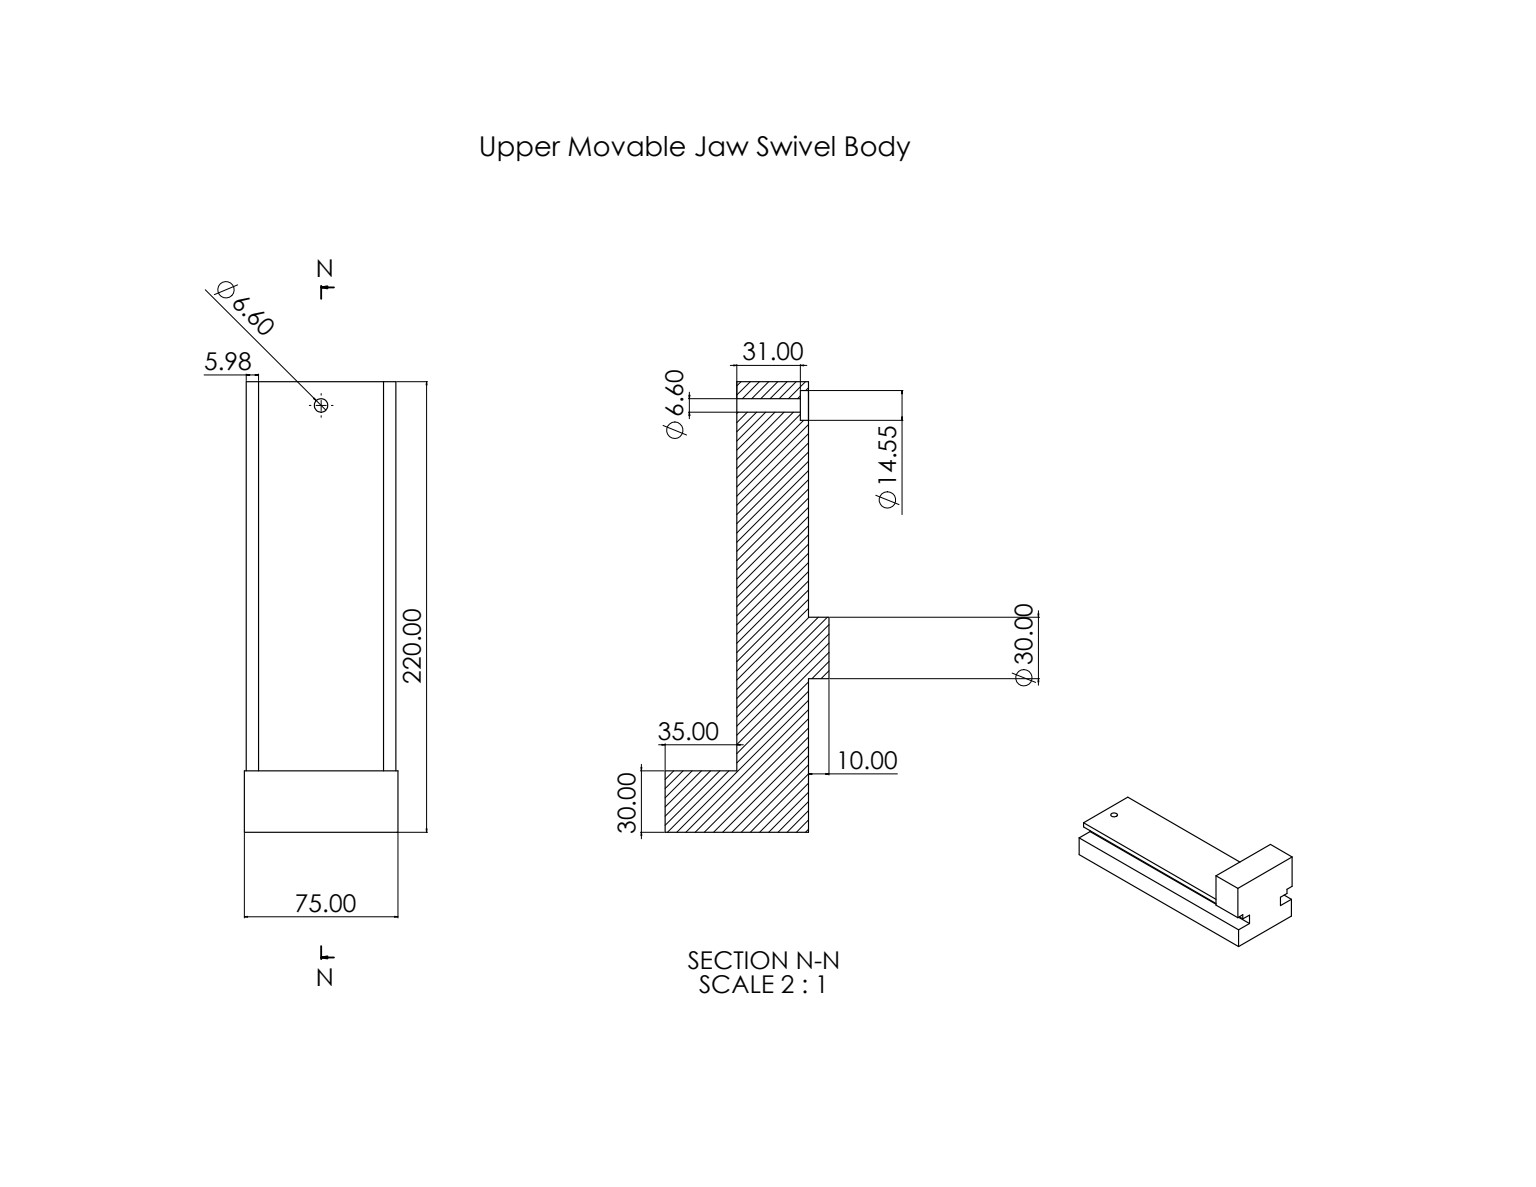
ISO-10303-21;
HEADER;
FILE_DESCRIPTION (('STEP AP214'),
    '1' );
FILE_NAME ('Upper Movable Jaw Swivel Body.step',
    '2026-10-24T22:31:37',
    ( '' ),
    ( '' ),
    'SwSTEP 2.0',
    'SolidWorks 2025',
    '' );
FILE_SCHEMA (( 'AUTOMOTIVE_DESIGN' ));
ENDSEC;

DATA;
#88=ORIENTED_EDGE ( 'NONE', *, *, #97854, .T. ) ;
#107=CARTESIAN_POINT ( 'NONE',  ( -32.94356256989595977, 94.88921800892812541, 10.61543114587583503 ) ) ;
#112=EDGE_CURVE ( 'NONE', #27867, #86369, #27228, .T. ) ;
#449=DIRECTION ( 'NONE',  ( 0.8660254037844391517, 0.4999999999999990008, 0.000000000000000000 ) ) ;
#471=DIRECTION ( 'NONE',  ( 0.8660254037844373753, 0.5000000000000021094, 0.000000000000000000 ) ) ;
#478=CARTESIAN_POINT ( 'NONE',  ( -32.68486601307109396, 95.73265939123938040, 11.22505256784756611 ) ) ;
#599=DIRECTION ( 'NONE',  ( 0.8660254037844382635, 0.5000000000000005551, 0.000000000000000000 ) ) ;
#606=VECTOR ( 'NONE', #83343, 1000.000000000000114 ) ;
#639=PLANE ( 'NONE',  #90141 ) ;
#678=( LENGTH_UNIT ( ) NAMED_UNIT ( * ) SI_UNIT ( .MILLI., .METRE. ) );
#987=ORIENTED_EDGE ( 'NONE', *, *, #63428, .F. ) ;
#1016=CARTESIAN_POINT ( 'NONE',  ( 77.93017357788673394, 184.0458036431182052, -30.52142883766498116 ) ) ;
#1096=DIRECTION ( 'NONE',  ( 0.000000000000000000, 0.000000000000000000, 1.000000000000000000 ) ) ;
#1182=DIRECTION ( 'NONE',  ( 0.8660254037844382635, 0.5000000000000005551, 0.000000000000000000 ) ) ;
#1406=VECTOR ( 'NONE', #11738, 1000.000000000000000 ) ;
#1495=ORIENTED_EDGE ( 'NONE', *, *, #73193, .T. ) ;
#1508=ORIENTED_EDGE ( 'NONE', *, *, #88243, .F. ) ;
#1527=ORIENTED_EDGE ( 'NONE', *, *, #76895, .F. ) ;
#1594=CARTESIAN_POINT ( 'NONE',  ( -167.0327448629461742, 42.61639673982678289, 21.50000000000000000 ) ) ;
#1831=ORIENTED_EDGE ( 'NONE', *, *, #24685, .F. ) ;
#2126=VERTEX_POINT ( 'NONE', #95140 ) ;
#2173=CARTESIAN_POINT ( 'NONE',  ( -132.5954152546898115, 108.6868197944956478, 37.50000000000002132 ) ) ;
#2180=DIRECTION ( 'NONE',  ( 1.000000000000000000, 0.000000000000000000, 0.000000000000000000 ) ) ;
#2356=CARTESIAN_POINT ( 'NONE',  ( -107.5954152546897262, 65.38554960527366688, -21.50000000000000000 ) ) ;
#2371=ORIENTED_EDGE ( 'NONE', *, *, #69900, .T. ) ;
#2442=CARTESIAN_POINT ( 'NONE',  ( -31.55997627504339320, 93.43085135866357405, 11.06573829301134282 ) ) ;
#2563=FACE_OUTER_BOUND ( 'NONE', #81678, .T. ) ;
#2588=EDGE_CURVE ( 'NONE', #83357, #20667, #32841, .T. ) ;
#2781=VECTOR ( 'NONE', #47717, 1000.000000000000227 ) ;
#2784=UNCERTAINTY_MEASURE_WITH_UNIT (LENGTH_MEASURE( 1.000000000000000082E-05 ), #94636, 'distance_accuracy_value', 'NONE');
#3036=VECTOR ( 'NONE', #61789, 1000.000000000000000 ) ;
#3092=ORIENTED_EDGE ( 'NONE', *, *, #37488, .F. ) ;
#3134=VECTOR ( 'NONE', #87868, 1000.000000000000000 ) ;
#3372=CARTESIAN_POINT ( 'NONE',  ( 65.36586985908989789, 182.5653022007868742, 0.000000000000000000 ) ) ;
#3536=DIRECTION ( 'NONE',  ( 0.5000000000000002220, -0.8660254037844387076, -0.000000000000000000 ) ) ;
#3607=CARTESIAN_POINT ( 'NONE',  ( -32.02765978341597730, 96.24804957567249630, 11.90709431551868214 ) ) ;
#3843=ORIENTED_EDGE ( 'NONE', *, *, #39130, .F. ) ;
#3870=ORIENTED_EDGE ( 'NONE', *, *, #76643, .F. ) ;
#3921=CARTESIAN_POINT ( 'NONE',  ( -32.85596848784926038, 94.38113866725780099, 10.43451941826970319 ) ) ;
#3932=ORIENTED_EDGE ( 'NONE', *, *, #2588, .T. ) ;
#4006=VECTOR ( 'NONE', #42693, 1000.000000000000000 ) ;
#4058=DIRECTION ( 'NONE',  ( 0.000000000000000000, 0.000000000000000000, -1.000000000000000000 ) ) ;
#4066=LINE ( 'NONE', #89237, #62676 ) ;
#4351=CARTESIAN_POINT ( 'NONE',  ( -14.30703472742949245, 105.2809231865207522, 10.47389102980036313 ) ) ;
#4594=LINE ( 'NONE', #12204, #86850 ) ;
#4680=CYLINDRICAL_SURFACE ( 'NONE', #36010, 3.300000000000010925 ) ;
#4830=VECTOR ( 'NONE', #48570, 1000.000000000000227 ) ;
#4863=ORIENTED_EDGE ( 'NONE', *, *, #15300, .T. ) ;
#4920=CARTESIAN_POINT ( 'NONE',  ( -13.86269525828469895, 104.2312461070084879, 10.61543114587583148 ) ) ;
#5067=FACE_OUTER_BOUND ( 'NONE', #46254, .T. ) ;
#5071=ORIENTED_EDGE ( 'NONE', *, *, #58498, .F. ) ;
#5089=DIRECTION ( 'NONE',  ( 0.8660254037844385966, 0.5000000000000001110, -0.000000000000000000 ) ) ;
#5122=LINE ( 'NONE', #90768, #6948 ) ;
#5352=CARTESIAN_POINT ( 'NONE',  ( -14.46602979551751389, 105.4129113170957481, 10.54689744722228006 ) ) ;
#5376=FACE_OUTER_BOUND ( 'NONE', #49831, .T. ) ;
#5390=VECTOR ( 'NONE', #56746, 1000.000000000000114 ) ;
#5468=ORIENTED_EDGE ( 'NONE', *, *, #67897, .F. ) ;
#5479=ADVANCED_FACE ( 'NONE', ( #20384 ), #4680, .F. ) ;
#5488=CARTESIAN_POINT ( 'NONE',  ( -167.0327448629461742, 42.61639673982678289, -21.50000000000000000 ) ) ;
#5508=CARTESIAN_POINT ( 'NONE',  ( 80.86586985908986946, 155.7185146834693512, 0.000000000000000000 ) ) ;
#5738=CARTESIAN_POINT ( 'NONE',  ( -14.65312891409034535, 84.40478749174073414, 0.000000000000000000 ) ) ;
#5800=FACE_OUTER_BOUND ( 'NONE', #65592, .T. ) ;
#5844=CARTESIAN_POINT ( 'NONE',  ( -16.76269525828470464, 104.2312461070085021, 12.63376007436041171 ) ) ;
#5851=DIRECTION ( 'NONE',  ( -0.000000000000000000, -0.000000000000000000, 1.000000000000000000 ) ) ;
#5871=PLANE ( 'NONE',  #22534 ) ;
#5896=ADVANCED_FACE ( 'NONE', ( #7535 ), #53628, .F. ) ;
#5923=ORIENTED_EDGE ( 'NONE', *, *, #44335, .T. ) ;
#5975=AXIS2_PLACEMENT_3D ( 'NONE', #18174, #69859, #471 ) ;
#6124=CIRCLE ( 'NONE', #70862, 7.273499999999997634 ) ;
#6152=FACE_OUTER_BOUND ( 'NONE', #19578, .T. ) ;
#6375=ADVANCED_FACE ( 'NONE', ( #54494 ), #23602, .T. ) ;
#6428=CONICAL_SURFACE ( 'NONE', #56528, 7.298499999999999766, 0.7853981633976494514 ) ;
#6948=VECTOR ( 'NONE', #7990, 1000.000000000000000 ) ;
#7015=ORIENTED_EDGE ( 'NONE', *, *, #33038, .F. ) ;
#7114=CARTESIAN_POINT ( 'NONE',  ( -97.59541525468981149, 48.06504152958505216, 36.50000000000000000 ) ) ;
#7240=VECTOR ( 'NONE', #599, 1000.000000000000114 ) ;
#7282=CARTESIAN_POINT ( 'NONE',  ( -27.64350997085663408, 76.90478749174087625, 0.000000000000000000 ) ) ;
#7348=VERTEX_POINT ( 'NONE', #39001 ) ;
#7439=ORIENTED_EDGE ( 'NONE', *, *, #88245, .T. ) ;
#7459=CARTESIAN_POINT ( 'NONE',  ( 82.93017357788667709, 175.3855496052738374, 36.50000000000000000 ) ) ;
#7460=DIRECTION ( 'NONE',  ( -0.000000000000000000, -0.000000000000000000, -1.000000000000000000 ) ) ;
#7523=ORIENTED_EDGE ( 'NONE', *, *, #37488, .T. ) ;
#7535=FACE_OUTER_BOUND ( 'NONE', #52527, .T. ) ;
#7609=LINE ( 'NONE', #1016, #16237 ) ;
#7691=DIRECTION ( 'NONE',  ( 0.5000000000000000000, -0.8660254037844387076, 0.000000000000000000 ) ) ;
#7767=VECTOR ( 'NONE', #54858, 1000.000000000000114 ) ;
#7861=EDGE_LOOP ( 'NONE', ( #9188, #92716, #77192, #81964 ) ) ;
#7990=DIRECTION ( 'NONE',  ( 0.4999999999999985012, -0.8660254037844394848, -1.387778780781440351E-15 ) ) ;
#8389=DIRECTION ( 'NONE',  ( -0.000000000000000000, -0.000000000000000000, 1.000000000000000000 ) ) ;
#8417=CARTESIAN_POINT ( 'NONE',  ( -89.11465314115667979, 93.37593066204033221, -30.52142883766496695 ) ) ;
#8555=CARTESIAN_POINT ( 'NONE',  ( 74.56683408466376761, 152.0817646834693448, 8.907468493598274475E-16 ) ) ;
#8757=LINE ( 'NONE', #2173, #11074 ) ;
#8809=ORIENTED_EDGE ( 'NONE', *, *, #62129, .T. ) ;
#8849=EDGE_LOOP ( 'NONE', ( #90481, #9070, #75347, #22436 ) ) ;
#8886=DIRECTION ( 'NONE',  ( -0.5000000000000003331, 0.8660254037844383745, 0.000000000000000000 ) ) ;
#8976=CARTESIAN_POINT ( 'NONE',  ( -106.6146531411566798, 123.6868197944956620, 37.50000000000002132 ) ) ;
#9070=ORIENTED_EDGE ( 'NONE', *, *, #32666, .F. ) ;
#9078=DIRECTION ( 'NONE',  ( 0.8660254037844384856, 0.5000000000000002220, 0.000000000000000000 ) ) ;
#9152=ORIENTED_EDGE ( 'NONE', *, *, #45013, .T. ) ;
#9188=ORIENTED_EDGE ( 'NONE', *, *, #12031, .F. ) ;
#9235=AXIS2_PLACEMENT_3D ( 'NONE', #17271, #24379, #9699 ) ;
#9406=ORIENTED_EDGE ( 'NONE', *, *, #12031, .T. ) ;
#9506=ADVANCED_FACE ( 'NONE', ( #29685 ), #76775, .T. ) ;
#9510=LINE ( 'NONE', #71312, #77599 ) ;
#9699=DIRECTION ( 'NONE',  ( 0.8660254037844373753, 0.5000000000000021094, 0.000000000000000000 ) ) ;
#9759=EDGE_CURVE ( 'NONE', #12458, #43772, #86395, .T. ) ;
#9788=CARTESIAN_POINT ( 'NONE',  ( -169.5327448629461742, 46.94652375874896677, 30.52142883766498827 ) ) ;
#9801=SHAPE_REPRESENTATION_RELATIONSHIP ( 'NONE' , 'NONE' ,  #87244, #17532 ) ;
#10026=CARTESIAN_POINT ( 'NONE',  ( 77.93017357788673394, 184.0458036431182052, 21.50000000000000000 ) ) ;
#10028=ORIENTED_EDGE ( 'NONE', *, *, #69900, .F. ) ;
#10091=DIRECTION ( 'NONE',  ( 0.5000000000000005551, -0.8660254037844382635, -3.965082230804119373E-16 ) ) ;
#10101=DIRECTION ( 'NONE',  ( 0.8660254037844382635, 0.5000000000000005551, 0.000000000000000000 ) ) ;
#10174=EDGE_CURVE ( 'NONE', #37839, #84449, #78305, .T. ) ;
#10179=DIRECTION ( 'NONE',  ( -0.8660254037844375974, -0.5000000000000016653, 0.000000000000000000 ) ) ;
#10198=EDGE_CURVE ( 'NONE', #33624, #79062, #80847, .T. ) ;
#10307=FACE_OUTER_BOUND ( 'NONE', #41949, .T. ) ;
#10553=ORIENTED_EDGE ( 'NONE', *, *, #33693, .T. ) ;
#10719=PLANE ( 'NONE',  #41218 ) ;
#10723=EDGE_LOOP ( 'NONE', ( #84176, #16172 ) ) ;
#10803=VERTEX_POINT ( 'NONE', #67448 ) ;
#10818=CARTESIAN_POINT ( 'NONE',  ( -107.5954152546898257, 65.38554960527383741, 36.50000000000000000 ) ) ;
#10849=ADVANCED_FACE ( 'NONE', ( #75563, #6152 ), #37045, .F. ) ;
#10855=CYLINDRICAL_SURFACE ( 'NONE', #91491, 14.99999999999968381 ) ;
#11014=VECTOR ( 'NONE', #31568, 1000.000000000000000 ) ;
#11074=VECTOR ( 'NONE', #17874, 1000.000000000000000 ) ;
#11139=DIRECTION ( 'NONE',  ( 0.5000000000000001110, -0.8660254037844384856, -0.000000000000000000 ) ) ;
#11216=CARTESIAN_POINT ( 'NONE',  ( -31.49991166888935368, 96.34225309604657639, 12.27547638658930218 ) ) ;
#11235=CARTESIAN_POINT ( 'NONE',  ( -167.0327448629461742, 42.61639673982675447, 30.52142883766498116 ) ) ;
#11374=AXIS2_PLACEMENT_3D ( 'NONE', #37260, #99085, #91499 ) ;
#11419=DIRECTION ( 'NONE',  ( -0.5000000000000002220, 0.8660254037844384856, 1.387778780781440548E-15 ) ) ;
#11527=CARTESIAN_POINT ( 'NONE',  ( -112.5954152546897120, 74.04580364311804885, -30.52142883766498116 ) ) ;
#11529=CARTESIAN_POINT ( 'NONE',  ( -16.75143828124104317, 104.0219442184326937, 12.69405866495271695 ) ) ;
#11540=CARTESIAN_POINT ( 'NONE',  ( -30.74734981195323158, 93.63450014558806345, 11.75270985346817909 ) ) ;
#11738=DIRECTION ( 'NONE',  ( -0.000000000000000000, -0.000000000000000000, 1.000000000000000000 ) ) ;
#11834=CARTESIAN_POINT ( 'NONE',  ( 82.93017357788673394, 175.3855496052738374, 21.50000000000000000 ) ) ;
#11858=CARTESIAN_POINT ( 'NONE',  ( 82.85336985908988083, 152.2760637034261890, 0.000000000000000000 ) ) ;
#11912=CARTESIAN_POINT ( 'NONE',  ( 76.55433408466377898, 148.6393137034262111, 8.907468493598274475E-16 ) ) ;
#11989=PRODUCT_DEFINITION_SHAPE ( 'NONE', 'NONE',  #32837 ) ;
#12018=CARTESIAN_POINT ( 'NONE',  ( -16.52110513491133759, 103.4226009623137514, 12.75654370805655091 ) ) ;
#12031=EDGE_CURVE ( 'NONE', #10803, #33624, #9510, .T. ) ;
#12050=CARTESIAN_POINT ( 'NONE',  ( 89.15240563351599690, 155.9128137034261954, 0.000000000000000000 ) ) ;
#12170=CARTESIAN_POINT ( 'NONE',  ( 82.93017357788673394, 175.3855496052738374, -21.50000000000000000 ) ) ;
#12198=CARTESIAN_POINT ( 'NONE',  ( -30.22813246154364109, 95.60533857986700923, 12.75846431767311451 ) ) ;
#12204=CARTESIAN_POINT ( 'NONE',  ( -89.11465314115667979, 93.37593066204033221, -30.52142883766496695 ) ) ;
#12217=DIRECTION ( 'NONE',  ( 0.000000000000000000, -1.000000000000000000, -1.201851678989722492E-15 ) ) ;
#12458=VERTEX_POINT ( 'NONE', #69665 ) ;
#12466=CARTESIAN_POINT ( 'NONE',  ( -15.24570502058241139, 105.6897125274499842, 11.06526020485377160 ) ) ;
#12473=CYLINDRICAL_SURFACE ( 'NONE', #44723, 1.449999999999993072 ) ;
#12517=CARTESIAN_POINT ( 'NONE',  ( -14.03049543618944206, 103.5316844796765565, 11.08926661400182390 ) ) ;
#12561=ORIENTED_EDGE ( 'NONE', *, *, #34818, .T. ) ;
#12682=DIRECTION ( 'NONE',  ( -0.5000000000000008882, 0.8660254037844381525, 0.000000000000000000 ) ) ;
#12687=AXIS2_PLACEMENT_3D ( 'NONE', #69833, #100261, #59733 ) ;
#12698=LINE ( 'NONE', #73992, #85196 ) ;
#12974=CARTESIAN_POINT ( 'NONE',  ( -15.07180212829954158, 105.6728077113080673, 10.93289567214266711 ) ) ;
#12998=CARTESIAN_POINT ( 'NONE',  ( -30.04356256989597185, 94.88921800892812541, 36.50000000000000000 ) ) ;
#13058=CARTESIAN_POINT ( 'NONE',  ( 87.16490563351598553, 159.3552646834693292, 0.000000000000000000 ) ) ;
#13093=EDGE_LOOP ( 'NONE', ( #90102, #1495, #15262, #82142 ) ) ;
#13128=LINE ( 'NONE', #14612, #83498 ) ;
#13202=CARTESIAN_POINT ( 'NONE',  ( -30.10073558955866702, 95.30624366923747459, 12.73418565006493175 ) ) ;
#13422=DIRECTION ( 'NONE',  ( 1.000000000000000000, 0.000000000000000000, 0.000000000000000000 ) ) ;
#13483=EDGE_LOOP ( 'NONE', ( #22501, #42882, #25014, #81312 ) ) ;
#13558=VECTOR ( 'NONE', #32477, 1000.000000000000114 ) ;
#13570=AXIS2_PLACEMENT_3D ( 'NONE', #14550, #53030, #65862 ) ;
#13616=DIRECTION ( 'NONE',  ( 0.5000000000000002220, -0.8660254037844387076, -0.000000000000000000 ) ) ;
#13794=ORIENTED_EDGE ( 'NONE', *, *, #88245, .F. ) ;
#14075=DIRECTION ( 'NONE',  ( 0.5000000000000006661, -0.8660254037844383745, -3.433594394091488070E-15 ) ) ;
#14147=VECTOR ( 'NONE', #8389, 1000.000000000000000 ) ;
#14187=CARTESIAN_POINT ( 'NONE',  ( -32.32883188359665638, 96.08671883726218255, 11.63744038197175534 ) ) ;
#14193=CARTESIAN_POINT ( 'NONE',  ( -32.94356256989595977, 94.88921800892812541, 36.50000000000000000 ) ) ;
#14304=AXIS2_PLACEMENT_3D ( 'NONE', #83231, #7691, #67996 ) ;
#14470=DIRECTION ( 'NONE',  ( 0.000000000000000000, 0.000000000000000000, 1.000000000000000000 ) ) ;
#14550=CARTESIAN_POINT ( 'NONE',  ( -15.31269525828471068, 104.2312461070085021, 36.50000000000000000 ) ) ;
#14566=EDGE_LOOP ( 'NONE', ( #92678, #83072, #30486, #36692 ) ) ;
#14612=CARTESIAN_POINT ( 'NONE',  ( -106.6146531411566798, 123.6868197944956620, 37.50000000000002132 ) ) ;
#14681=CARTESIAN_POINT ( 'NONE',  ( -32.77609386396424185, 95.58753423100951352, 11.08839328151203851 ) ) ;
#14906=ORIENTED_EDGE ( 'NONE', *, *, #33038, .T. ) ;
#15085=DIRECTION ( 'NONE',  ( 0.000000000000000000, -0.000000000000000000, 1.000000000000000000 ) ) ;
#15251=LINE ( 'NONE', #1594, #13558 ) ;
#15262=ORIENTED_EDGE ( 'NONE', *, *, #99216, .F. ) ;
#15267=CARTESIAN_POINT ( 'NONE',  ( 0.000000000000000000, 0.000000000000000000, -36.50000000000000000 ) ) ;
#15300=EDGE_CURVE ( 'NONE', #94383, #88861, #37826, .T. ) ;
#15314=ADVANCED_FACE ( 'NONE', ( #37879 ), #22709, .T. ) ;
#15354=CARTESIAN_POINT ( 'NONE',  ( 0.000000000000000000, 0.000000000000000000, 0.000000000000000000 ) ) ;
#15546=PLANE ( 'NONE',  #96769 ) ;
#15668=ORIENTED_EDGE ( 'NONE', *, *, #91252, .F. ) ;
#15713=CYLINDRICAL_SURFACE ( 'NONE', #61431, 1.449999999999993072 ) ;
#15866=AXIS2_PLACEMENT_3D ( 'NONE', #15267, #1096, #69484 ) ;
#15879=VECTOR ( 'NONE', #30098, 999.9999999999998863 ) ;
#15919=VECTOR ( 'NONE', #98723, 1000.000000000000000 ) ;
#16027=ORIENTED_EDGE ( 'NONE', *, *, #57557, .F. ) ;
#16172=ORIENTED_EDGE ( 'NONE', *, *, #9759, .T. ) ;
#16182=VECTOR ( 'NONE', #99200, 1000.000000000000114 ) ;
#16237=VECTOR ( 'NONE', #47103, 1000.000000000000114 ) ;
#16312=CARTESIAN_POINT ( 'NONE',  ( -1.662747857324051282, 91.90478749174060624, 1.836970198720990540E-15 ) ) ;
#16329=LINE ( 'NONE', #78145, #88768 ) ;
#16549=CARTESIAN_POINT ( 'NONE',  ( -169.5327448629461742, 46.94652375874896677, 30.52142883766498827 ) ) ;
#16698=ORIENTED_EDGE ( 'NONE', *, *, #50936, .F. ) ;
#16721=EDGE_CURVE ( 'NONE', #7348, #56899, #5122, .T. ) ;
#16855=VECTOR ( 'NONE', #32280, 1000.000000000000114 ) ;
#16871=LINE ( 'NONE', #40156, #51977 ) ;
#17082=ADVANCED_FACE ( 'NONE', ( #44850 ), #61041, .T. ) ;
#17173=ORIENTED_EDGE ( 'NONE', *, *, #45138, .F. ) ;
#17200=VECTOR ( 'NONE', #22885, 1000.000000000000000 ) ;
#17265=ORIENTED_EDGE ( 'NONE', *, *, #17424, .T. ) ;
#17271=CARTESIAN_POINT ( 'NONE',  ( 80.86586985908986946, 155.7185146834693512, 0.000000000000000000 ) ) ;
#17365=ADVANCED_FACE ( 'NONE', ( #62930 ), #639, .T. ) ;
#17424=EDGE_CURVE ( 'NONE', #27867, #82530, #25430, .T. ) ;
#17532=ADVANCED_BREP_SHAPE_REPRESENTATION ( '', ( #77374, #68784 ), #36458 ) ;
#17765=CARTESIAN_POINT ( 'NONE',  ( -167.0327448629461742, 42.61639673982678289, -21.50000000000000000 ) ) ;
#17787=EDGE_LOOP ( 'NONE', ( #74842, #9152, #46683, #35102 ) ) ;
#17874=DIRECTION ( 'NONE',  ( -7.401486830834377265E-16, 7.401486830834377265E-16, -1.000000000000000000 ) ) ;
#17933=AXIS2_PLACEMENT_3D ( 'NONE', #67594, #82850, #74235 ) ;
#18128=CARTESIAN_POINT ( 'NONE',  ( -30.04356256989558815, 94.88921800892795488, 12.63376007436073323 ) ) ;
#18174=CARTESIAN_POINT ( 'NONE',  ( 80.86586985908986946, 155.7185146834693512, 0.000000000000000000 ) ) ;
#18282=EDGE_CURVE ( 'NONE', #99384, #50939, #27437, .T. ) ;
#18412=ORIENTED_EDGE ( 'NONE', *, *, #86727, .F. ) ;
#18517=EDGE_CURVE ( 'NONE', #23627, #46799, #73912, .T. ) ;
#18560=DIRECTION ( 'NONE',  ( -1.982541115402060426E-16, 3.433861939970638790E-16, -1.000000000000000000 ) ) ;
#18566=DIRECTION ( 'NONE',  ( 0.8660254037844377084, 0.5000000000000016653, 0.000000000000000000 ) ) ;
#18568=CARTESIAN_POINT ( 'NONE',  ( -16.56403295706242318, 104.9882471913986990, 12.26538863783448186 ) ) ;
#18579=ORIENTED_EDGE ( 'NONE', *, *, #93323, .T. ) ;
#18690=ORIENTED_EDGE ( 'NONE', *, *, #57557, .T. ) ;
#18827=APPLICATION_CONTEXT ( 'automotive_design' ) ;
#18886=CARTESIAN_POINT ( 'NONE',  ( -13.86269525828469895, 104.2312461070084879, 10.61543114587583148 ) ) ;
#18947=LINE ( 'NONE', #49826, #33470 ) ;
#19147=CARTESIAN_POINT ( 'NONE',  ( -30.24407882362163846, 94.12867598954146331, 12.26304263616266077 ) ) ;
#19442=ORIENTED_EDGE ( 'NONE', *, *, #68029, .F. ) ;
#19531=ORIENTED_EDGE ( 'NONE', *, *, #89878, .F. ) ;
#19560=DIRECTION ( 'NONE',  ( 0.5000000000000001110, -0.8660254037844384856, -0.000000000000000000 ) ) ;
#19578=EDGE_LOOP ( 'NONE', ( #4863, #88 ) ) ;
#19581=CARTESIAN_POINT ( 'NONE',  ( -14.23124088391897146, 105.2031859152619120, 10.44627079400605218 ) ) ;
#19596=EDGE_CURVE ( 'NONE', #91708, #27867, #13128, .T. ) ;
#19632=CARTESIAN_POINT ( 'NONE',  ( -16.31118285231257303, 103.1745050122371481, 12.72070314857826467 ) ) ;
#19643=CARTESIAN_POINT ( 'NONE',  ( -30.60512737934784155, 93.72946926685976621, 11.88605707516453691 ) ) ;
#19824=ORIENTED_EDGE ( 'NONE', *, *, #67897, .T. ) ;
#19825=CARTESIAN_POINT ( 'NONE',  ( 82.93017357788667709, 175.3855496052738374, 36.50000000000000000 ) ) ;
#19890=DIRECTION ( 'NONE',  ( 0.8660254037844373753, 0.5000000000000021094, 0.000000000000000000 ) ) ;
#19964=VERTEX_POINT ( 'NONE', #44378 ) ;
#20066=CARTESIAN_POINT ( 'NONE',  ( -14.55094619507370801, 105.4688078659398514, 10.59293022331821099 ) ) ;
#20069=DIRECTION ( 'NONE',  ( -0.8660254037844382635, -0.5000000000000004441, 0.000000000000000000 ) ) ;
#20118=CARTESIAN_POINT ( 'NONE',  ( -14.76680962501131589, 102.8402364515597469, 11.91671626263131856 ) ) ;
#20129=CARTESIAN_POINT ( 'NONE',  ( -32.26013835757641601, 93.64104699330448511, 10.58366280279360971 ) ) ;
#20179=DIRECTION ( 'NONE',  ( 0.5000000000000014433, -0.8660254037844379305, 0.000000000000000000 ) ) ;
#20243=DIRECTION ( 'NONE',  ( 0.8660254037844391517, 0.4999999999999990008, 0.000000000000000000 ) ) ;
#20307=ORIENTED_EDGE ( 'NONE', *, *, #86286, .T. ) ;
#20384=FACE_OUTER_BOUND ( 'NONE', #17787, .T. ) ;
#20667=VERTEX_POINT ( 'NONE', #58531 ) ;
#20988=EDGE_CURVE ( 'NONE', #84449, #47085, #84745, .T. ) ;
#21072=ORIENTED_EDGE ( 'NONE', *, *, #77053, .T. ) ;
#21291=LINE ( 'NONE', #35969, #67737 ) ;
#21354=EDGE_CURVE ( 'NONE', #62277, #32844, #96223, .T. ) ;
#21790=AXIS2_PLACEMENT_3D ( 'NONE', #73940, #67832, #20243 ) ;
#21893=LINE ( 'NONE', #98918, #17200 ) ;
#22006=ORIENTED_EDGE ( 'NONE', *, *, #21354, .F. ) ;
#22032=CARTESIAN_POINT ( 'NONE',  ( -16.76269525828470464, 104.4383445782105042, 12.56748295067274945 ) ) ;
#22180=VECTOR ( 'NONE', #42070, 1000.000000000000114 ) ;
#22397=ORIENTED_EDGE ( 'NONE', *, *, #41041, .F. ) ;
#22436=ORIENTED_EDGE ( 'NONE', *, *, #95215, .T. ) ;
#22501=ORIENTED_EDGE ( 'NONE', *, *, #23408, .F. ) ;
#22522=VECTOR ( 'NONE', #62854, 1000.000000000000000 ) ;
#22526=VECTOR ( 'NONE', #1182, 1000.000000000000114 ) ;
#22534=AXIS2_PLACEMENT_3D ( 'NONE', #98595, #14470, #68652 ) ;
#22639=EDGE_LOOP ( 'NONE', ( #58236, #64858, #7523, #3843 ) ) ;
#22709=PLANE ( 'NONE',  #89665 ) ;
#22835=EDGE_CURVE ( 'NONE', #85740, #37839, #63017, .T. ) ;
#22880=FACE_OUTER_BOUND ( 'NONE', #67161, .T. ) ;
#22885=DIRECTION ( 'NONE',  ( -0.2588190451027150840, -0.9659258262890161317, 8.659560562356675748E-17 ) ) ;
#22966=( NAMED_UNIT ( * ) SI_UNIT ( $, .STERADIAN. ) SOLID_ANGLE_UNIT ( ) );
#23131=CARTESIAN_POINT ( 'NONE',  ( -89.11465314115662295, 93.37593066204024694, -30.52142883766498116 ) ) ;
#23363=EDGE_LOOP ( 'NONE', ( #18412, #51644, #99432, #18690 ) ) ;
#23373=LINE ( 'NONE', #77608, #70923 ) ;
#23390=CARTESIAN_POINT ( 'NONE',  ( 82.93017357788667709, 175.3855496052738374, 36.50000000000000000 ) ) ;
#23408=EDGE_CURVE ( 'NONE', #98986, #24620, #81400, .T. ) ;
#23457=DIRECTION ( 'NONE',  ( 1.000000000000000000, 0.000000000000000000, 0.000000000000000000 ) ) ;
#23602=PLANE ( 'NONE',  #67693 ) ;
#23608=EDGE_LOOP ( 'NONE', ( #8809, #13794, #86714, #37581, #78724, #9406, #80355, #86475, #67151, #79423, #31254, #86823, #5923, #41180, #92068, #80132 ) ) ;
#23627=VERTEX_POINT ( 'NONE', #89514 ) ;
#23629=CARTESIAN_POINT ( 'NONE',  ( 62.50798602660126591, 180.9153022007868685, 4.041334437186263538E-16 ) ) ;
#23630=ADVANCED_FACE ( 'NONE', ( #81896 ), #12473, .F. ) ;
#23875=PLANE ( 'NONE',  #15866 ) ;
#23896=DIRECTION ( 'NONE',  ( -0.8660254037844385966, -0.4999999999999999445, 0.000000000000000000 ) ) ;
#23972=VERTEX_POINT ( 'NONE', #34847 ) ;
#24157=PLANE ( 'NONE',  #43501 ) ;
#24326=DIRECTION ( 'NONE',  ( 0.5000000000000000000, -0.8660254037844387076, 0.000000000000000000 ) ) ;
#24373=ORIENTED_EDGE ( 'NONE', *, *, #40599, .F. ) ;
#24379=DIRECTION ( 'NONE',  ( 0.5000000000000002220, -0.8660254037844387076, -0.000000000000000000 ) ) ;
#24447=EDGE_LOOP ( 'NONE', ( #93056, #65035 ) ) ;
#24486=AXIS2_PLACEMENT_3D ( 'NONE', #99117, #29699, #45388 ) ;
#24620=VERTEX_POINT ( 'NONE', #81268 ) ;
#24685=EDGE_CURVE ( 'NONE', #67744, #41262, #18947, .T. ) ;
#24700=CARTESIAN_POINT ( 'NONE',  ( -89.11465314115665137, 93.37593066204027537, 37.50000000000002132 ) ) ;
#24766=PLANE ( 'NONE',  #43274 ) ;
#24982=ORIENTED_EDGE ( 'NONE', *, *, #29271, .F. ) ;
#25014=ORIENTED_EDGE ( 'NONE', *, *, #41013, .F. ) ;
#25049=PRODUCT_DEFINITION_CONTEXT ( 'detailed design', #54587, 'design' ) ;
#25103=ORIENTED_EDGE ( 'NONE', *, *, #86286, .F. ) ;
#25219=CARTESIAN_POINT ( 'NONE',  ( -97.59541525468981149, 48.06504152958505216, 36.50000000000000000 ) ) ;
#25232=ORIENTED_EDGE ( 'NONE', *, *, #59302, .F. ) ;
#25430=LINE ( 'NONE', #47230, #2781 ) ;
#25626=ADVANCED_FACE ( 'NONE', ( #50332 ), #10855, .T. ) ;
#25654=CIRCLE ( 'NONE', #48349, 3.299999999999998934 ) ;
#25739=CARTESIAN_POINT ( 'NONE',  ( -32.76508427577140736, 94.18386203199597162, 10.41389758979254587 ) ) ;
#25748=ORIENTED_EDGE ( 'NONE', *, *, #94596, .F. ) ;
#26009=ORIENTED_EDGE ( 'NONE', *, *, #34192, .T. ) ;
#26014=DIRECTION ( 'NONE',  ( 0.5000000000000001110, -0.8660254037844385966, 0.000000000000000000 ) ) ;
#26521=VERTEX_POINT ( 'NONE', #46463 ) ;
#26564=FACE_OUTER_BOUND ( 'NONE', #46792, .T. ) ;
#26953=CARTESIAN_POINT ( 'NONE',  ( -107.5954152546898257, 65.38554960527383741, -21.50000000000000000 ) ) ;
#27228=LINE ( 'NONE', #41405, #92812 ) ;
#27229=CARTESIAN_POINT ( 'NONE',  ( -32.94356256989596687, 94.79146141117595903, 10.56663419031904638 ) ) ;
#27437=LINE ( 'NONE', #81173, #1406 ) ;
#27607=ORIENTED_EDGE ( 'NONE', *, *, #83276, .T. ) ;
#27638=ORIENTED_EDGE ( 'NONE', *, *, #39847, .F. ) ;
#27645=LINE ( 'NONE', #35724, #48129 ) ;
#27666=CARTESIAN_POINT ( 'NONE',  ( -13.95001416935992289, 104.7385778355855592, 10.43465946748403184 ) ) ;
#27867=VERTEX_POINT ( 'NONE', #89401 ) ;
#27902=ORIENTED_EDGE ( 'NONE', *, *, #34818, .F. ) ;
#28141=CARTESIAN_POINT ( 'NONE',  ( 83.72375369157853697, 157.3685146834693569, 0.000000000000000000 ) ) ;
#28296=DIRECTION ( 'NONE',  ( 0.8660254037844390407, 0.4999999999999993339, 0.000000000000000000 ) ) ;
#28683=DIRECTION ( 'NONE',  ( 0.8660254037844384856, 0.5000000000000002220, 0.000000000000000000 ) ) ;
#28818=EDGE_CURVE ( 'NONE', #88861, #86378, #12698, .T. ) ;
#28890=CARTESIAN_POINT ( 'NONE',  ( -31.21596018254677674, 96.31576462380481018, 12.43553956882932354 ) ) ;
#28906=VECTOR ( 'NONE', #99966, 1000.000000000000227 ) ;
#28970=CARTESIAN_POINT ( 'NONE',  ( 92.93017357788669131, 158.0650415295850735, 36.50000000000000000 ) ) ;
#28997=EDGE_LOOP ( 'NONE', ( #5071, #94941, #48935, #1508 ) ) ;
#29099=CARTESIAN_POINT ( 'NONE',  ( 82.93017357788673394, 175.3855496052738374, 21.50000000000000000 ) ) ;
#29127=VERTEX_POINT ( 'NONE', #31360 ) ;
#29271=EDGE_CURVE ( 'NONE', #45307, #72476, #86890, .T. ) ;
#29349=VERTEX_POINT ( 'NONE', #23131 ) ;
#29622=ORIENTED_EDGE ( 'NONE', *, *, #97854, .F. ) ;
#29626=VERTEX_POINT ( 'NONE', #93846 ) ;
#29685=FACE_OUTER_BOUND ( 'NONE', #14566, .T. ) ;
#29699=DIRECTION ( 'NONE',  ( 0.5000000000000002220, -0.8660254037844387076, -0.000000000000000000 ) ) ;
#29771=LINE ( 'NONE', #7459, #44943 ) ;
#29833=EDGE_LOOP ( 'NONE', ( #5468, #88382, #20307, #987 ) ) ;
#29897=DIRECTION ( 'NONE',  ( 1.000000000000000000, 0.000000000000000000, 0.000000000000000000 ) ) ;
#29909=ORIENTED_EDGE ( 'NONE', *, *, #66198, .F. ) ;
#30098=DIRECTION ( 'NONE',  ( -0.5000000000000014433, 0.8660254037844379305, -0.000000000000000000 ) ) ;
#30375=LINE ( 'NONE', #92228, #68159 ) ;
#30486=ORIENTED_EDGE ( 'NONE', *, *, #85239, .T. ) ;
#30520=CARTESIAN_POINT ( 'NONE',  ( -16.76269525828470464, 104.2312461070085021, 36.50000000000000000 ) ) ;
#30568=B_SPLINE_CURVE_WITH_KNOTS ( 'NONE', 3,
 ( #50672, #82644, #65879, #13202, #73015, #12198, #36471, #65386, #81625, #67375, #98301, #28890, #59768, #11216, #34485, #42083, #3607, #14187, #61261, #478, #14681, #37955, #69373, #60257 ),
 .UNSPECIFIED., .F., .F.,
 ( 4, 2, 2, 2, 2, 2, 2, 2, 2, 2, 2, 4 ),
 ( 1.437624280391282253E-16, 0.0003245379161388591786, 0.0006490758322775745919, 0.0009736137484162901137, 0.001298151664555005419, 0.001947227496832436462, 0.002271765412971152309, 0.002596303329109868590, 0.003245379161387301151, 0.003894454993664734146, 0.004543530825942166708, 0.005192606658219600137 ),
 .UNSPECIFIED. ) ;
#30592=LINE ( 'NONE', #77183, #11014 ) ;
#30691=CARTESIAN_POINT ( 'NONE',  ( -13.86269525828471849, 104.2312461070085021, 45.19948692389422717 ) ) ;
#30697=CARTESIAN_POINT ( 'NONE',  ( 92.93017357788669131, 158.0650415295850735, 36.50000000000000000 ) ) ;
#30790=CARTESIAN_POINT ( 'NONE',  ( 82.93017357788667709, 175.3855496052738374, -36.50000000000000000 ) ) ;
#30901=CARTESIAN_POINT ( 'NONE',  ( 75.43017357788674815, 188.3759306620403891, 30.52142883766498827 ) ) ;
#30973=EDGE_CURVE ( 'NONE', #43772, #20667, #93009, .T. ) ;
#31062=ORIENTED_EDGE ( 'NONE', *, *, #98811, .T. ) ;
#31149=EDGE_CURVE ( 'NONE', #89481, #41262, #33521, .T. ) ;
#31254=ORIENTED_EDGE ( 'NONE', *, *, #50987, .T. ) ;
#31333=ADVANCED_FACE ( 'NONE', ( #68271 ), #51584, .T. ) ;
#31360=CARTESIAN_POINT ( 'NONE',  ( -132.5954152546898115, 108.6868197944956478, 37.50000000000002132 ) ) ;
#31403=B_SPLINE_CURVE_WITH_KNOTS ( 'NONE', 3,
 ( #96600, #89985, #51441, #49954, #27666, #89032, #80911, #19581, #4351, #5352, #20066, #35246, #58534, #12974, #12466, #43835, #36233, #98061, #57036, #88019, #18568, #75759, #22032, #5844 ),
 .UNSPECIFIED., .F., .F.,
 ( 4, 2, 2, 2, 2, 2, 2, 2, 2, 2, 2, 4 ),
 ( 1.440969542111313559E-17, 0.0003279589196580527753, 0.0006559178393160911306, 0.0009838767589741292691, 0.001311835678632167733, 0.001639794598290206197, 0.001967753517948244227, 0.002623671357264322455, 0.003279589196580400684, 0.003935507035896478045, 0.004591424875212556274, 0.005247342714528634502 ),
 .UNSPECIFIED. ) ;
#31432=DIRECTION ( 'NONE',  ( 0.9659258262891203817, -0.2588190451023261174, 0.000000000000000000 ) ) ;
#31454=VECTOR ( 'NONE', #35297, 1000.000000000000114 ) ;
#31568=DIRECTION ( 'NONE',  ( -0.000000000000000000, -0.000000000000000000, -1.000000000000000000 ) ) ;
#31714=LINE ( 'NONE', #2356, #52905 ) ;
#31719=FACE_OUTER_BOUND ( 'NONE', #86164, .T. ) ;
#31732=CARTESIAN_POINT ( 'NONE',  ( -27.64350997085663764, 76.90478749174087625, 0.000000000000000000 ) ) ;
#31986=ORIENTED_EDGE ( 'NONE', *, *, #73526, .T. ) ;
#32005=ORIENTED_EDGE ( 'NONE', *, *, #98306, .F. ) ;
#32191=ORIENTED_EDGE ( 'NONE', *, *, #20988, .T. ) ;
#32216=CARTESIAN_POINT ( 'NONE',  ( -167.0327448629461742, 42.61639673982678289, -30.52142883766498116 ) ) ;
#32280=DIRECTION ( 'NONE',  ( 0.8660254037844382635, 0.5000000000000005551, 0.000000000000000000 ) ) ;
#32282=CARTESIAN_POINT ( 'NONE',  ( -89.11465314115665137, 93.37593066204027537, 37.50000000000002132 ) ) ;
#32411=ADVANCED_FACE ( 'NONE', ( #55645 ), #24766, .T. ) ;
#32430=DIRECTION ( 'NONE',  ( -0.000000000000000000, -0.000000000000000000, 1.000000000000000000 ) ) ;
#32477=DIRECTION ( 'NONE',  ( 0.8660254037844382635, 0.5000000000000005551, 0.000000000000000000 ) ) ;
#32492=VERTEX_POINT ( 'NONE', #23629 ) ;
#32500=DIRECTION ( 'NONE',  ( -0.5000000000000001110, 0.8660254037844385966, 0.000000000000000000 ) ) ;
#32598=PLANE ( 'NONE',  #61293 ) ;
#32666=EDGE_CURVE ( 'NONE', #43772, #12458, #31403, .T. ) ;
#32837=PRODUCT_DEFINITION ( 'UNKNOWN', '', #52713, #25049 ) ;
#32841=CIRCLE ( 'NONE', #89533, 1.449999999999993072 ) ;
#32844=VERTEX_POINT ( 'NONE', #48597 ) ;
#32875=CARTESIAN_POINT ( 'NONE',  ( -115.0954152546897973, 78.37593066204027537, -37.49999999999999289 ) ) ;
#32986=CARTESIAN_POINT ( 'NONE',  ( -115.0954152546900673, 78.37593066204081538, 30.52142883766498827 ) ) ;
#32991=AXIS2_PLACEMENT_3D ( 'NONE', #5508, #13616, #28296 ) ;
#32997=ADVANCED_FACE ( 'NONE', ( #52070 ), #15546, .T. ) ;
#33038=EDGE_CURVE ( 'NONE', #84449, #86487, #29771, .T. ) ;
#33077=DIRECTION ( 'NONE',  ( -0.5000000000000001110, 0.8660254037844385966, 0.000000000000000000 ) ) ;
#33448=EDGE_LOOP ( 'NONE', ( #27638, #27902 ) ) ;
#33470=VECTOR ( 'NONE', #80783, 1000.000000000000114 ) ;
#33521=LINE ( 'NONE', #19825, #91848 ) ;
#33607=DIRECTION ( 'NONE',  ( -0.8660254037844385966, -0.5000000000000001110, -6.091690621058838765E-17 ) ) ;
#33624=VERTEX_POINT ( 'NONE', #85273 ) ;
#33693=EDGE_CURVE ( 'NONE', #29349, #26521, #16329, .T. ) ;
#33897=CARTESIAN_POINT ( 'NONE',  ( -89.11465314115667979, 93.37593066204033221, -30.52142883766496695 ) ) ;
#34148=ADVANCED_FACE ( 'NONE', ( #22880 ), #23875, .F. ) ;
#34192=EDGE_CURVE ( 'NONE', #23972, #45307, #23373, .T. ) ;
#34320=CARTESIAN_POINT ( 'NONE',  ( -32.70769541684651216, 94.08906143139476796, 10.41629251971181702 ) ) ;
#34339=ORIENTED_EDGE ( 'NONE', *, *, #24685, .T. ) ;
#34381=EDGE_CURVE ( 'NONE', #73648, #67744, #21291, .T. ) ;
#34485=CARTESIAN_POINT ( 'NONE',  ( -31.59167490957833735, 96.33871916006887659, 12.21808272424466502 ) ) ;
#34662=VECTOR ( 'NONE', #56131, 1000.000000000000000 ) ;
#34734=DIRECTION ( 'NONE',  ( -0.5000000000000005551, 0.8660254037844384856, 0.000000000000000000 ) ) ;
#34796=ADVANCED_FACE ( 'NONE', ( #31719 ), #55518, .T. ) ;
#34802=DIRECTION ( 'NONE',  ( 0.5000000000000005551, -0.8660254037844382635, -3.965082230804119373E-16 ) ) ;
#34803=CARTESIAN_POINT ( 'NONE',  ( -30.05514682052448450, 94.68088024134054592, 12.56018961544704915 ) ) ;
#34818=EDGE_CURVE ( 'NONE', #32492, #23972, #41839, .T. ) ;
#34847=CARTESIAN_POINT ( 'NONE',  ( 68.22375369157856539, 184.2153022007868799, 0.000000000000000000 ) ) ;
#34937=CARTESIAN_POINT ( 'NONE',  ( -112.5954152546897262, 74.04580364311806306, -30.52142883766498116 ) ) ;
#34948=PLANE ( 'NONE',  #40109 ) ;
#34951=CARTESIAN_POINT ( 'NONE',  ( -14.65312891409034535, 84.40478749174073414, 0.000000000000000000 ) ) ;
#34959=LINE ( 'NONE', #73985, #22180 ) ;
#34969=AXIS2_PLACEMENT_3D ( 'NONE', #55423, #55921, #78265 ) ;
#35010=CARTESIAN_POINT ( 'NONE',  ( 92.93017357788669131, 158.0650415295850735, -36.50000000000000000 ) ) ;
#35064=CARTESIAN_POINT ( 'NONE',  ( 82.86586985908988368, 152.2544130683315871, 0.000000000000000000 ) ) ;
#35102=ORIENTED_EDGE ( 'NONE', *, *, #34192, .F. ) ;
#35246=CARTESIAN_POINT ( 'NONE',  ( -14.72174178882247908, 105.5588735921874672, 10.69508629217443207 ) ) ;
#35251=DIRECTION ( 'NONE',  ( 0.000000000000000000, 0.000000000000000000, 1.000000000000000000 ) ) ;
#35297=DIRECTION ( 'NONE',  ( 0.5000000000000002220, -0.8660254037844384856, 0.000000000000000000 ) ) ;
#35298=CARTESIAN_POINT ( 'NONE',  ( -15.49448615033923815, 102.7791273954868672, 12.38876935695490822 ) ) ;
#35358=FACE_OUTER_BOUND ( 'NONE', #24447, .T. ) ;
#35474=VECTOR ( 'NONE', #10101, 1000.000000000000114 ) ;
#35482=DIRECTION ( 'NONE',  ( 0.8660254037844377084, 0.5000000000000016653, 0.000000000000000000 ) ) ;
#35636=DIRECTION ( 'NONE',  ( 0.5000000000000001110, -0.8660254037844387076, -0.000000000000000000 ) ) ;
#35724=CARTESIAN_POINT ( 'NONE',  ( -97.59541525468981149, 48.06504152958505216, -36.50000000000000000 ) ) ;
#35792=CARTESIAN_POINT ( 'NONE',  ( -6.662747857324019307, 100.5650415295849029, 1.836970198720990540E-15 ) ) ;
#35969=CARTESIAN_POINT ( 'NONE',  ( 92.93017357788669131, 158.0650415295850735, -36.50000000000000000 ) ) ;
#36010=AXIS2_PLACEMENT_3D ( 'NONE', #35064, #57868, #19890 ) ;
#36188=CYLINDRICAL_SURFACE ( 'NONE', #17933, 3.300000000000010925 ) ;
#36233=CARTESIAN_POINT ( 'NONE',  ( -15.75121124376761905, 105.6236688776997710, 11.47872565613448614 ) ) ;
#36235=LINE ( 'NONE', #45810, #99710 ) ;
#36458=( GEOMETRIC_REPRESENTATION_CONTEXT ( 3 ) GLOBAL_UNCERTAINTY_ASSIGNED_CONTEXT ( ( #93996 ) ) GLOBAL_UNIT_ASSIGNED_CONTEXT ( ( #678, #38152, #22966 ) ) REPRESENTATION_CONTEXT ( 'NONE', 'WORKASPACE' ) );
#36471=CARTESIAN_POINT ( 'NONE',  ( -30.28621228554850831, 95.69946231200637499, 12.75647095971420697 ) ) ;
#36656=ORIENTED_EDGE ( 'NONE', *, *, #41013, .T. ) ;
#36692=ORIENTED_EDGE ( 'NONE', *, *, #54036, .T. ) ;
#36723=ORIENTED_EDGE ( 'NONE', *, *, #82786, .F. ) ;
#36735=DIRECTION ( 'NONE',  ( 1.000000000000000000, 0.000000000000000000, 0.000000000000000000 ) ) ;
#36756=FACE_BOUND ( 'NONE', #39541, .T. ) ;
#36777=CARTESIAN_POINT ( 'NONE',  ( -89.11465314115667979, 93.37593066204033221, -30.52142883766496695 ) ) ;
#36854=EDGE_LOOP ( 'NONE', ( #41671, #16027, #96193, #17265 ) ) ;
#37045=PLANE ( 'NONE',  #40328 ) ;
#37051=DIRECTION ( 'NONE',  ( -0.000000000000000000, -0.000000000000000000, -1.000000000000000000 ) ) ;
#37092=FACE_OUTER_BOUND ( 'NONE', #48091, .T. ) ;
#37193=DIRECTION ( 'NONE',  ( 0.000000000000000000, 0.000000000000000000, 1.000000000000000000 ) ) ;
#37260=CARTESIAN_POINT ( 'NONE',  ( -31.49356256989596758, 94.88921800892812541, 45.19948692389422717 ) ) ;
#37340=ORIENTED_EDGE ( 'NONE', *, *, #22835, .F. ) ;
#37354=VECTOR ( 'NONE', #97899, 1000.000000000000000 ) ;
#37488=EDGE_CURVE ( 'NONE', #2126, #7348, #55832, .T. ) ;
#37581=ORIENTED_EDGE ( 'NONE', *, *, #90907, .T. ) ;
#37826=CIRCLE ( 'NONE', #32991, 7.273499999999997634 ) ;
#37839=VERTEX_POINT ( 'NONE', #79084 ) ;
#37879=FACE_OUTER_BOUND ( 'NONE', #13093, .T. ) ;
#37919=VERTEX_POINT ( 'NONE', #49151 ) ;
#37955=CARTESIAN_POINT ( 'NONE',  ( -32.90453922033355383, 95.26561800654556578, 10.83411691445564351 ) ) ;
#37998=DIRECTION ( 'NONE',  ( 0.8660254037844385966, 0.5000000000000003331, -0.000000000000000000 ) ) ;
#38152=( NAMED_UNIT ( * ) PLANE_ANGLE_UNIT ( ) SI_UNIT ( $, .RADIAN. ) );
#38284=AXIS2_PLACEMENT_3D ( 'NONE', #34951, #71981, #10179 ) ;
#38456=DIRECTION ( 'NONE',  ( -0.5000000000000002220, 0.8660254037844384856, 0.000000000000000000 ) ) ;
#38505=FACE_OUTER_BOUND ( 'NONE', #23608, .T. ) ;
#38644=AXIS2_PLACEMENT_3D ( 'NONE', #11858, #89400, #98453 ) ;
#38825=DIRECTION ( 'NONE',  ( 0.5000000000000002220, -0.8660254037844384856, 0.000000000000000000 ) ) ;
#39001=CARTESIAN_POINT ( 'NONE',  ( 75.43017357788674815, 188.3759306620403891, 30.52142883766498827 ) ) ;
#39130=EDGE_CURVE ( 'NONE', #26521, #7348, #54176, .T. ) ;
#39157=LINE ( 'NONE', #7282, #59486 ) ;
#39541=EDGE_LOOP ( 'NONE', ( #97706, #67975 ) ) ;
#39660=EDGE_LOOP ( 'NONE', ( #77356, #78518, #31986, #21072 ) ) ;
#39847=EDGE_CURVE ( 'NONE', #23972, #32492, #25654, .T. ) ;
#40102=MECHANICAL_DESIGN_GEOMETRIC_PRESENTATION_REPRESENTATION('',(#85513),#96784);
#40109=AXIS2_PLACEMENT_3D ( 'NONE', #67348, #4058, #74975 ) ;
#40156=CARTESIAN_POINT ( 'NONE',  ( -115.0954152546897973, 78.37593066204027537, 37.50000000000002132 ) ) ;
#40328=AXIS2_PLACEMENT_3D ( 'NONE', #67953, #99859, #53244 ) ;
#40599=EDGE_CURVE ( 'NONE', #91566, #50040, #50004, .T. ) ;
#40998=CIRCLE ( 'NONE', #13570, 1.449999999999993072 ) ;
#41013=EDGE_CURVE ( 'NONE', #91836, #77883, #54746, .T. ) ;
#41041=EDGE_CURVE ( 'NONE', #89481, #91836, #65847, .T. ) ;
#41071=ORIENTED_EDGE ( 'NONE', *, *, #94596, .T. ) ;
#41180=ORIENTED_EDGE ( 'NONE', *, *, #23408, .T. ) ;
#41218=AXIS2_PLACEMENT_3D ( 'NONE', #11235, #81646, #12217 ) ;
#41234=CYLINDRICAL_SURFACE ( 'NONE', #80318, 14.99999999999968381 ) ;
#41262=VERTEX_POINT ( 'NONE', #43524 ) ;
#41269=CARTESIAN_POINT ( 'NONE',  ( -112.5954152546897120, 74.04580364311802043, 30.52142883766498116 ) ) ;
#41405=CARTESIAN_POINT ( 'NONE',  ( -89.11465314115665137, 93.37593066204027537, -37.49999999999999289 ) ) ;
#41627=AXIS2_PLACEMENT_3D ( 'NONE', #60769, #82664, #29897 ) ;
#41671=ORIENTED_EDGE ( 'NONE', *, *, #77669, .F. ) ;
#41839=CIRCLE ( 'NONE', #95266, 3.299999999999998934 ) ;
#41895=AXIS2_PLACEMENT_3D ( 'NONE', #73653, #35636, #89402 ) ;
#41901=CARTESIAN_POINT ( 'NONE',  ( -16.76269525828470464, 104.1287493039388181, 12.66656182927058261 ) ) ;
#41910=DIRECTION ( 'NONE',  ( -1.538313725856140942E-15, 3.076627451712281884E-15, -1.000000000000000000 ) ) ;
#41949=EDGE_LOOP ( 'NONE', ( #16698, #68541, #70135, #19531, #84328, #29909 ) ) ;
#42070=DIRECTION ( 'NONE',  ( 0.8660254037844382635, 0.5000000000000005551, 0.000000000000000000 ) ) ;
#42083=CARTESIAN_POINT ( 'NONE',  ( -31.86071352217370034, 96.30357957927230927, 12.03701289477871761 ) ) ;
#42226=DIRECTION ( 'NONE',  ( -0.5000000000000014433, 0.8660254037844378194, -0.000000000000000000 ) ) ;
#42341=AXIS2_PLACEMENT_3D ( 'NONE', #94779, #72474, #63841 ) ;
#42531=DIRECTION ( 'NONE',  ( 0.5000000000000001110, -0.8660254037844384856, -0.000000000000000000 ) ) ;
#42693=DIRECTION ( 'NONE',  ( 0.5000000000000008882, -0.8660254037844381525, -0.000000000000000000 ) ) ;
#42828=DIRECTION ( 'NONE',  ( -0.5000000000000005551, 0.8660254037844383745, 0.000000000000000000 ) ) ;
#42846=EDGE_CURVE ( 'NONE', #10803, #37919, #15251, .T. ) ;
#42882=ORIENTED_EDGE ( 'NONE', *, *, #60365, .T. ) ;
#43056=VERTEX_POINT ( 'NONE', #51672 ) ;
#43082=DIRECTION ( 'NONE',  ( -0.000000000000000000, -0.000000000000000000, -1.000000000000000000 ) ) ;
#43259=ORIENTED_EDGE ( 'NONE', *, *, #73526, .F. ) ;
#43274=AXIS2_PLACEMENT_3D ( 'NONE', #33897, #86138, #9078 ) ;
#43288=CIRCLE ( 'NONE', #72552, 1.449999999999993072 ) ;
#43389=CARTESIAN_POINT ( 'NONE',  ( -13.90044561320711480, 103.8584542157411761, 10.83137812414022605 ) ) ;
#43470=CARTESIAN_POINT ( 'NONE',  ( -107.5954152546897404, 65.38554960527368110, 21.50000000000000000 ) ) ;
#43501=AXIS2_PLACEMENT_3D ( 'NONE', #16549, #42828, #20069 ) ;
#43524=CARTESIAN_POINT ( 'NONE',  ( 82.93017357788667709, 175.3855496052738374, -36.50000000000000000 ) ) ;
#43772=VERTEX_POINT ( 'NONE', #18886 ) ;
#43835=CARTESIAN_POINT ( 'NONE',  ( -15.58608437336083696, 105.6654254483952826, 11.33858688303593709 ) ) ;
#44225=DIRECTION ( 'NONE',  ( -0.5000000000000014433, 0.8660254037844378194, -0.000000000000000000 ) ) ;
#44314=ORIENTED_EDGE ( 'NONE', *, *, #20988, .F. ) ;
#44335=EDGE_CURVE ( 'NONE', #46799, #98986, #80963, .T. ) ;
#44378=CARTESIAN_POINT ( 'NONE',  ( -89.11465314115665137, 93.37593066204027537, 37.50000000000002132 ) ) ;
#44647=ORIENTED_EDGE ( 'NONE', *, *, #58580, .T. ) ;
#44723=AXIS2_PLACEMENT_3D ( 'NONE', #91475, #5851, #36735 ) ;
#44850=FACE_OUTER_BOUND ( 'NONE', #10723, .T. ) ;
#44894=EDGE_CURVE ( 'NONE', #33624, #56899, #63687, .T. ) ;
#44943=VECTOR ( 'NONE', #46967, 1000.000000000000000 ) ;
#44945=VECTOR ( 'NONE', #31432, 1000.000000000000000 ) ;
#44968=VERTEX_POINT ( 'NONE', #46990 ) ;
#45013=EDGE_CURVE ( 'NONE', #32492, #72476, #65315, .T. ) ;
#45120=FACE_OUTER_BOUND ( 'NONE', #98697, .T. ) ;
#45138=EDGE_CURVE ( 'NONE', #91866, #56834, #94639, .T. ) ;
#45307=VERTEX_POINT ( 'NONE', #28141 ) ;
#45388=DIRECTION ( 'NONE',  ( 0.8660254037844391517, 0.4999999999999990008, 0.000000000000000000 ) ) ;
#45603=PLANE ( 'NONE',  #65669 ) ;
#45810=CARTESIAN_POINT ( 'NONE',  ( -30.04356256989597185, 94.88921800892812541, 45.19948692389422717 ) ) ;
#45817=ORIENTED_EDGE ( 'NONE', *, *, #93824, .T. ) ;
#45883=ADVANCED_FACE ( 'NONE', ( #64916 ), #10719, .T. ) ;
#46254=EDGE_LOOP ( 'NONE', ( #98527, #45817, #22397, #19442 ) ) ;
#46463=CARTESIAN_POINT ( 'NONE',  ( 75.43017357788674815, 188.3759306620403891, -30.52142883766498116 ) ) ;
#46683=ORIENTED_EDGE ( 'NONE', *, *, #60251, .T. ) ;
#46792=EDGE_LOOP ( 'NONE', ( #1527, #17173, #71752, #50234 ) ) ;
#46799=VERTEX_POINT ( 'NONE', #47788 ) ;
#46967=DIRECTION ( 'NONE',  ( -0.000000000000000000, -0.000000000000000000, -1.000000000000000000 ) ) ;
#46990=CARTESIAN_POINT ( 'NONE',  ( 76.54518344956915143, 148.6051630683315921, 8.938084663576969700E-16 ) ) ;
#47085=VERTEX_POINT ( 'NONE', #10818 ) ;
#47103=DIRECTION ( 'NONE',  ( -0.4999999999999987788, 0.8660254037844392627, 0.000000000000000000 ) ) ;
#47230=CARTESIAN_POINT ( 'NONE',  ( -106.6146531411567224, 123.6868197944957188, -37.49999999999997868 ) ) ;
#47300=ORIENTED_EDGE ( 'NONE', *, *, #31149, .T. ) ;
#47440=EDGE_LOOP ( 'NONE', ( #32005, #25103 ) ) ;
#47552=CARTESIAN_POINT ( 'NONE',  ( 89.16490563351598553, 155.8911630683315934, 0.000000000000000000 ) ) ;
#47651=AXIS2_PLACEMENT_3D ( 'NONE', #95609, #57034, #18566 ) ;
#47717=DIRECTION ( 'NONE',  ( -0.8660254037844384856, -0.5000000000000002220, 0.000000000000000000 ) ) ;
#47788=CARTESIAN_POINT ( 'NONE',  ( -115.0954152546898257, 78.37593066204033221, -30.52142883766498116 ) ) ;
#47933=VECTOR ( 'NONE', #48997, 1000.000000000000227 ) ;
#47971=LINE ( 'NONE', #32282, #47933 ) ;
#48091=EDGE_LOOP ( 'NONE', ( #22006, #53496, #47300, #53256 ) ) ;
#48119=ORIENTED_EDGE ( 'NONE', *, *, #28818, .T. ) ;
#48129=VECTOR ( 'NONE', #19560, 1000.000000000000227 ) ;
#48349=AXIS2_PLACEMENT_3D ( 'NONE', #60644, #91600, #53064 ) ;
#48361=EDGE_LOOP ( 'NONE', ( #79135, #41071, #10553, #49089, #63987 ) ) ;
#48534=LINE ( 'NONE', #25219, #81018 ) ;
#48570=DIRECTION ( 'NONE',  ( 0.5000000000000001110, -0.8660254037844384856, -0.000000000000000000 ) ) ;
#48597=CARTESIAN_POINT ( 'NONE',  ( -107.5954152546898257, 65.38554960527383741, -36.50000000000000000 ) ) ;
#48935=ORIENTED_EDGE ( 'NONE', *, *, #60007, .T. ) ;
#48997=DIRECTION ( 'NONE',  ( -0.8660254037844384856, -0.5000000000000002220, 0.000000000000000000 ) ) ;
#49029=CARTESIAN_POINT ( 'NONE',  ( -32.89006047420026135, 94.48531712824750173, 10.45786326575769998 ) ) ;
#49089=ORIENTED_EDGE ( 'NONE', *, *, #83276, .F. ) ;
#49151=CARTESIAN_POINT ( 'NONE',  ( 77.93017357788673394, 184.0458036431182052, 21.50000000000000000 ) ) ;
#49495=ADVANCED_FACE ( 'NONE', ( #38505 ), #45603, .F. ) ;
#49826=CARTESIAN_POINT ( 'NONE',  ( 92.93017357788669131, 158.0650415295850735, -36.50000000000000000 ) ) ;
#49831=EDGE_LOOP ( 'NONE', ( #83219, #32191, #59604, #87303 ) ) ;
#49954=CARTESIAN_POINT ( 'NONE',  ( -13.91626742945881468, 104.6355682312461113, 10.45771055378636660 ) ) ;
#50004=CIRCLE ( 'NONE', #41895, 14.99999999999968026 ) ;
#50008=CARTESIAN_POINT ( 'NONE',  ( -16.70556162152145774, 103.8144583182831298, 12.73413235864565785 ) ) ;
#50021=CARTESIAN_POINT ( 'NONE',  ( -30.12762649812272997, 94.39323202455672401, 12.42295412654578435 ) ) ;
#50040=VERTEX_POINT ( 'NONE', #35792 ) ;
#50149=CARTESIAN_POINT ( 'NONE',  ( 82.86586985908988368, 152.2544130683315871, 0.000000000000000000 ) ) ;
#50164=CYLINDRICAL_SURFACE ( 'NONE', #38284, 14.99999999999968381 ) ;
#50234=ORIENTED_EDGE ( 'NONE', *, *, #40599, .T. ) ;
#50308=LINE ( 'NONE', #11834, #4006 ) ;
#50332=FACE_OUTER_BOUND ( 'NONE', #28997, .T. ) ;
#50465=ORIENTED_EDGE ( 'NONE', *, *, #44894, .T. ) ;
#50492=CARTESIAN_POINT ( 'NONE',  ( -15.87523210145152674, 102.8908870699714697, 12.57042221494010903 ) ) ;
#50504=CARTESIAN_POINT ( 'NONE',  ( -31.73672677518723972, 93.44825184473781121, 10.93130056797209981 ) ) ;
#50672=CARTESIAN_POINT ( 'NONE',  ( -30.04356256989558815, 94.88921800892795488, 12.63376007436073323 ) ) ;
#50749=ADVANCED_FACE ( 'NONE', ( #35358 ), #65752, .T. ) ;
#50928=AXIS2_PLACEMENT_3D ( 'NONE', #50149, #42531, #73464 ) ;
#50936=EDGE_CURVE ( 'NONE', #86369, #29349, #4594, .T. ) ;
#50939=VERTEX_POINT ( 'NONE', #14193 ) ;
#50987=EDGE_CURVE ( 'NONE', #82530, #23627, #71400, .T. ) ;
#50989=CARTESIAN_POINT ( 'NONE',  ( -14.45613220355349426, 103.0143348366940046, 11.63587646907208573 ) ) ;
#51441=CARTESIAN_POINT ( 'NONE',  ( -13.87263394856965704, 104.4305210064043052, 10.52386804011639221 ) ) ;
#51584=PLANE ( 'NONE',  #54540 ) ;
#51644=ORIENTED_EDGE ( 'NONE', *, *, #54036, .F. ) ;
#51672=CARTESIAN_POINT ( 'NONE',  ( 89.18655626861058749, 155.9036630683315821, 0.000000000000000000 ) ) ;
#51936=ADVANCED_FACE ( 'NONE', ( #97288 ), #99812, .F. ) ;
#51977=VECTOR ( 'NONE', #33077, 1000.000000000000000 ) ;
#52070=FACE_OUTER_BOUND ( 'NONE', #7861, .T. ) ;
#52400=LINE ( 'NONE', #74741, #606 ) ;
#52527=EDGE_LOOP ( 'NONE', ( #29622, #48119, #19824, #43259 ) ) ;
#52672=VERTEX_POINT ( 'NONE', #43470 ) ;
#52713=PRODUCT_DEFINITION_FORMATION_WITH_SPECIFIED_SOURCE ( 'ANY', '', #89683, .NOT_KNOWN. ) ;
#52859=VECTOR ( 'NONE', #10091, 1000.000000000000227 ) ;
#52905=VECTOR ( 'NONE', #38825, 1000.000000000000114 ) ;
#52921=DIRECTION ( 'NONE',  ( 0.8660254037844385966, 0.5000000000000001110, -0.000000000000000000 ) ) ;
#53030=DIRECTION ( 'NONE',  ( 0.000000000000000000, 0.000000000000000000, 1.000000000000000000 ) ) ;
#53064=DIRECTION ( 'NONE',  ( -0.8660254037844363761, -0.5000000000000039968, 0.000000000000000000 ) ) ;
#53244=DIRECTION ( 'NONE',  ( -0.8660254037844384856, -0.5000000000000001110, 0.000000000000000000 ) ) ;
#53256=ORIENTED_EDGE ( 'NONE', *, *, #82786, .T. ) ;
#53286=DIRECTION ( 'NONE',  ( 0.5000000000000001110, -0.8660254037844384856, -0.000000000000000000 ) ) ;
#53316=CARTESIAN_POINT ( 'NONE',  ( -162.0327448629461742, 33.95614270198240803, -21.50000000000000000 ) ) ;
#53458=ADVANCED_FACE ( 'NONE', ( #26564 ), #41234, .T. ) ;
#53496=ORIENTED_EDGE ( 'NONE', *, *, #68029, .T. ) ;
#53628=CYLINDRICAL_SURFACE ( 'NONE', #12687, 7.273499999999997634 ) ;
#54036=EDGE_CURVE ( 'NONE', #19964, #57005, #47971, .T. ) ;
#54176=LINE ( 'NONE', #30901, #3036 ) ;
#54202=CARTESIAN_POINT ( 'NONE',  ( -132.5954152546898683, 108.6868197944957046, -37.49999999999997868 ) ) ;
#54310=CARTESIAN_POINT ( 'NONE',  ( -89.11465314115665137, 93.37593066204027537, 37.50000000000002132 ) ) ;
#54403=CIRCLE ( 'NONE', #34969, 14.99999999999968026 ) ;
#54455=EDGE_CURVE ( 'NONE', #86378, #44968, #21893, .T. ) ;
#54494=FACE_OUTER_BOUND ( 'NONE', #48361, .T. ) ;
#54540=AXIS2_PLACEMENT_3D ( 'NONE', #5488, #99194, #59152 ) ;
#54587=APPLICATION_CONTEXT ( 'automotive_design' ) ;
#54622=DIRECTION ( 'NONE',  ( 0.5000000000000001110, -0.8660254037844384856, -0.000000000000000000 ) ) ;
#54746=LINE ( 'NONE', #87741, #22522 ) ;
#54780=FACE_BOUND ( 'NONE', #91746, .T. ) ;
#54787=LINE ( 'NONE', #62890, #7240 ) ;
#54858=DIRECTION ( 'NONE',  ( 0.8660254037844382635, 0.5000000000000005551, 0.000000000000000000 ) ) ;
#55268=PLANE ( 'NONE',  #95193 ) ;
#55423=CARTESIAN_POINT ( 'NONE',  ( -19.65312891409032403, 93.06504152958505927, 0.000000000000000000 ) ) ;
#55518=PLANE ( 'NONE',  #66146 ) ;
#55564=CARTESIAN_POINT ( 'NONE',  ( -167.0327448629461742, 42.61639673982675447, 30.52142883766498116 ) ) ;
#55582=DIRECTION ( 'NONE',  ( -0.5000000000000001110, 0.8660254037844385966, 0.000000000000000000 ) ) ;
#55645=FACE_OUTER_BOUND ( 'NONE', #57537, .T. ) ;
#55715=LINE ( 'NONE', #61335, #44945 ) ;
#55760=FACE_OUTER_BOUND ( 'NONE', #78470, .T. ) ;
#55832=LINE ( 'NONE', #9788, #7767 ) ;
#55921=DIRECTION ( 'NONE',  ( 0.5000000000000001110, -0.8660254037844387076, -0.000000000000000000 ) ) ;
#56083=LINE ( 'NONE', #24700, #70939 ) ;
#56106=DIRECTION ( 'NONE',  ( 0.5000000000000001110, -0.8660254037844384856, -0.000000000000000000 ) ) ;
#56131=DIRECTION ( 'NONE',  ( -3.977257660627182967E-15, 7.954515321254365934E-15, 1.000000000000000000 ) ) ;
#56197=CARTESIAN_POINT ( 'NONE',  ( 82.85336985908988083, 152.2760637034261890, 0.000000000000000000 ) ) ;
#56238=LINE ( 'NONE', #17765, #5390 ) ;
#56409=DIRECTION ( 'NONE',  ( 0.8660254037844390407, 0.4999999999999993339, 0.000000000000000000 ) ) ;
#56528=AXIS2_PLACEMENT_3D ( 'NONE', #94186, #54622, #449 ) ;
#56618=CARTESIAN_POINT ( 'NONE',  ( -32.08474812827099498, 93.55280042723998690, 10.69171554455069284 ) ) ;
#56746=DIRECTION ( 'NONE',  ( 0.8660254037844382635, 0.5000000000000005551, 0.000000000000000000 ) ) ;
#56834=VERTEX_POINT ( 'NONE', #16312 ) ;
#56851=CARTESIAN_POINT ( 'NONE',  ( -15.31269525828471068, 104.2312461070085021, 36.50000000000000000 ) ) ;
#56858=CARTESIAN_POINT ( 'NONE',  ( -162.0327448629461742, 33.95614270198240803, 21.50000000000000000 ) ) ;
#56899=VERTEX_POINT ( 'NONE', #70508 ) ;
#57005=VERTEX_POINT ( 'NONE', #89277 ) ;
#57034=DIRECTION ( 'NONE',  ( 0.5000000000000014433, -0.8660254037844379305, 0.000000000000000000 ) ) ;
#57036=CARTESIAN_POINT ( 'NONE',  ( -16.20514820903670028, 105.3874431953180135, 11.89003404754207160 ) ) ;
#57229=CYLINDRICAL_SURFACE ( 'NONE', #42341, 1.449999999999993072 ) ;
#57238=FACE_OUTER_BOUND ( 'NONE', #39660, .T. ) ;
#57358=AXIS2_PLACEMENT_3D ( 'NONE', #72134, #63012, #56409 ) ;
#57537=EDGE_LOOP ( 'NONE', ( #86650, #25748, #73492, #10028 ) ) ;
#57557=EDGE_CURVE ( 'NONE', #91708, #29127, #4066, .T. ) ;
#57868=DIRECTION ( 'NONE',  ( 0.5000000000000001110, -0.8660254037844384856, -0.000000000000000000 ) ) ;
#57904=ORIENTED_EDGE ( 'NONE', *, *, #18282, .F. ) ;
#58101=CARTESIAN_POINT ( 'NONE',  ( -16.67133665550712962, 103.7130579026488988, 12.74716765046184896 ) ) ;
#58236=ORIENTED_EDGE ( 'NONE', *, *, #33693, .F. ) ;
#58386=EDGE_LOOP ( 'NONE', ( #98400, #86231, #88632, #100051 ) ) ;
#58423=DIRECTION ( 'NONE',  ( -0.8660254037844375974, -0.5000000000000016653, 0.000000000000000000 ) ) ;
#58498=EDGE_CURVE ( 'NONE', #56834, #91866, #64358, .T. ) ;
#58511=PLANE ( 'NONE',  #67513 ) ;
#58531=CARTESIAN_POINT ( 'NONE',  ( -13.86269525828471849, 104.2312461070085021, 36.50000000000000000 ) ) ;
#58534=CARTESIAN_POINT ( 'NONE',  ( -14.80832225825293946, 105.5937860941667736, 10.75146334683068972 ) ) ;
#58580=EDGE_CURVE ( 'NONE', #29626, #99384, #30568, .T. ) ;
#58594=CARTESIAN_POINT ( 'NONE',  ( -30.04356256989597895, 94.78415495659865542, 12.60013705013512819 ) ) ;
#58778=CLOSED_SHELL ( 'NONE', ( #25626, #51936, #5896, #5479, #83177, #82515, #23630, #87689, #79528, #68882, #62176, #78872, #49495, #64910, #68368, #34148, #15314, #32997, #45883, #6375, #31333, #88629, #9506, #32411, #34796, #70340, #17365, #80228, #84872, #10849, #99041, #81917, #50749, #53458, #61264, #17082 ) ) ;
#59152=DIRECTION ( 'NONE',  ( 0.8660254037844382635, 0.5000000000000005551, 0.000000000000000000 ) ) ;
#59241=ORIENTED_EDGE ( 'NONE', *, *, #30973, .F. ) ;
#59267=DIRECTION ( 'NONE',  ( -0.000000000000000000, -0.000000000000000000, -1.000000000000000000 ) ) ;
#59302=EDGE_CURVE ( 'NONE', #29626, #68532, #36235, .T. ) ;
#59366=ORIENTED_EDGE ( 'NONE', *, *, #93323, .F. ) ;
#59486=VECTOR ( 'NONE', #100007, 999.9999999999998863 ) ;
#59500=DIRECTION ( 'NONE',  ( 0.5000000000000004441, -0.8660254037844383745, 0.000000000000000000 ) ) ;
#59604=ORIENTED_EDGE ( 'NONE', *, *, #74787, .T. ) ;
#59733=DIRECTION ( 'NONE',  ( 0.8660254037844390407, 0.4999999999999993339, 0.000000000000000000 ) ) ;
#59763=ORIENTED_EDGE ( 'NONE', *, *, #98811, .F. ) ;
#59768=CARTESIAN_POINT ( 'NONE',  ( -31.31209261750204931, 96.33089062496601684, 12.38423361974427372 ) ) ;
#59888=PLANE ( 'NONE',  #14304 ) ;
#59914=ORIENTED_EDGE ( 'NONE', *, *, #34381, .F. ) ;
#59926=ORIENTED_EDGE ( 'NONE', *, *, #16721, .T. ) ;
#59999=ORIENTED_EDGE ( 'NONE', *, *, #91252, .T. ) ;
#60007=EDGE_CURVE ( 'NONE', #50040, #91566, #54403, .T. ) ;
#60048=FACE_OUTER_BOUND ( 'NONE', #94584, .T. ) ;
#60251=EDGE_CURVE ( 'NONE', #72476, #45307, #60916, .T. ) ;
#60257=CARTESIAN_POINT ( 'NONE',  ( -32.94356256989595977, 94.88921800892812541, 10.61543114587583503 ) ) ;
#60365=EDGE_CURVE ( 'NONE', #98986, #77883, #34959, .T. ) ;
#60644=CARTESIAN_POINT ( 'NONE',  ( 65.36586985908989789, 182.5653022007868742, 0.000000000000000000 ) ) ;
#60756=DIRECTION ( 'NONE',  ( 4.546899780356472071E-16, -9.093799560712944142E-16, 1.000000000000000000 ) ) ;
#60769=CARTESIAN_POINT ( 'NONE',  ( -31.49356256989596758, 94.88921800892812541, 36.50000000000000000 ) ) ;
#60829=PRODUCT_CONTEXT ( 'NONE', #18827, 'mechanical' ) ;
#60916=CIRCLE ( 'NONE', #9235, 3.300000000000010925 ) ;
#61041=CYLINDRICAL_SURFACE ( 'NONE', #77146, 14.99999999999968381 ) ;
#61063=EDGE_CURVE ( 'NONE', #24620, #62277, #31714, .T. ) ;
#61261=CARTESIAN_POINT ( 'NONE',  ( -32.46101061832366952, 95.98221459296189551, 11.49967512814420445 ) ) ;
#61264=ADVANCED_FACE ( 'NONE', ( #73976 ), #50164, .T. ) ;
#61293=AXIS2_PLACEMENT_3D ( 'NONE', #78210, #33607, #26014 ) ;
#61335=CARTESIAN_POINT ( 'NONE',  ( 89.18655626861060171, 155.9036630683315821, 0.000000000000000000 ) ) ;
#61431=AXIS2_PLACEMENT_3D ( 'NONE', #99843, #32430, #63325 ) ;
#61789=DIRECTION ( 'NONE',  ( -0.000000000000000000, -0.000000000000000000, 1.000000000000000000 ) ) ;
#61918=DIRECTION ( 'NONE',  ( 0.000000000000000000, 0.000000000000000000, 1.000000000000000000 ) ) ;
#62129=EDGE_CURVE ( 'NONE', #32844, #73648, #27645, .T. ) ;
#62176=ADVANCED_FACE ( 'NONE', ( #66622 ), #58511, .F. ) ;
#62277=VERTEX_POINT ( 'NONE', #26953 ) ;
#62369=VECTOR ( 'NONE', #7460, 1000.000000000000000 ) ;
#62470=LINE ( 'NONE', #72115, #3134 ) ;
#62676=VECTOR ( 'NONE', #66857, 1000.000000000000227 ) ;
#62837=PLANE ( 'NONE',  #90411 ) ;
#62854=DIRECTION ( 'NONE',  ( 0.000000000000000000, 0.000000000000000000, -1.000000000000000000 ) ) ;
#62882=CARTESIAN_POINT ( 'NONE',  ( 92.93017357788669131, 158.0650415295850735, 36.50000000000000000 ) ) ;
#62890=CARTESIAN_POINT ( 'NONE',  ( -169.5327448629461742, 46.94652375874896677, 30.52142883766498827 ) ) ;
#62930=FACE_OUTER_BOUND ( 'NONE', #23363, .T. ) ;
#62938=CARTESIAN_POINT ( 'NONE',  ( -89.11465314115665137, 93.37593066204027537, -37.49999999999999289 ) ) ;
#62977=VECTOR ( 'NONE', #8886, 1000.000000000000114 ) ;
#63012=DIRECTION ( 'NONE',  ( 0.5000000000000002220, -0.8660254037844387076, -0.000000000000000000 ) ) ;
#63017=LINE ( 'NONE', #85367, #75422 ) ;
#63175=CARTESIAN_POINT ( 'NONE',  ( -32.64350997085663408, 85.56504152958521559, 0.000000000000000000 ) ) ;
#63245=FACE_OUTER_BOUND ( 'NONE', #58386, .T. ) ;
#63325=DIRECTION ( 'NONE',  ( 1.000000000000000000, 0.000000000000000000, 0.000000000000000000 ) ) ;
#63428=EDGE_CURVE ( 'NONE', #94311, #43056, #55715, .T. ) ;
#63687=LINE ( 'NONE', #55564, #16855 ) ;
#63841=DIRECTION ( 'NONE',  ( 1.000000000000000000, 0.000000000000000000, 0.000000000000000000 ) ) ;
#63968=ORIENTED_EDGE ( 'NONE', *, *, #99216, .T. ) ;
#63987=ORIENTED_EDGE ( 'NONE', *, *, #60365, .F. ) ;
#64070=ORIENTED_EDGE ( 'NONE', *, *, #34381, .T. ) ;
#64282=CIRCLE ( 'NONE', #41627, 1.449999999999993072 ) ;
#64347=CARTESIAN_POINT ( 'NONE',  ( -106.6146531411566798, 123.6868197944956620, 37.50000000000002132 ) ) ;
#64358=CIRCLE ( 'NONE', #90293, 14.99999999999968381 ) ;
#64732=CARTESIAN_POINT ( 'NONE',  ( -30.35047437581953034, 93.97944682170771102, 12.14429053135152792 ) ) ;
#64823=DIRECTION ( 'NONE',  ( 0.8660254037844390407, 0.4999999999999993339, 0.000000000000000000 ) ) ;
#64858=ORIENTED_EDGE ( 'NONE', *, *, #66198, .T. ) ;
#64910=ADVANCED_FACE ( 'NONE', ( #54780, #77086, #55760 ), #55268, .F. ) ;
#64916=FACE_OUTER_BOUND ( 'NONE', #75260, .T. ) ;
#65001=LINE ( 'NONE', #88356, #37354 ) ;
#65035=ORIENTED_EDGE ( 'NONE', *, *, #58498, .T. ) ;
#65036=ORIENTED_EDGE ( 'NONE', *, *, #50987, .F. ) ;
#65147=ORIENTED_EDGE ( 'NONE', *, *, #60251, .F. ) ;
#65207=CARTESIAN_POINT ( 'NONE',  ( -16.14732403980535835, 103.0408369278337801, 12.67348291615926215 ) ) ;
#65218=CARTESIAN_POINT ( 'NONE',  ( -32.49964441091157141, 93.83990077386336282, 10.47370245339621420 ) ) ;
#65246=ORIENTED_EDGE ( 'NONE', *, *, #29271, .T. ) ;
#65266=EDGE_LOOP ( 'NONE', ( #24982, #65147 ) ) ;
#65315=LINE ( 'NONE', #96254, #70221 ) ;
#65349=CYLINDRICAL_SURFACE ( 'NONE', #50928, 7.273499999999997634 ) ;
#65356=DIRECTION ( 'NONE',  ( 0.5000000000000001110, -0.8660254037844384856, -0.000000000000000000 ) ) ;
#65386=CARTESIAN_POINT ( 'NONE',  ( -30.41973204483513982, 95.86956414332775012, 12.73750267444827422 ) ) ;
#65592=EDGE_LOOP ( 'NONE', ( #73474, #12561, #26009, #65246 ) ) ;
#65669=AXIS2_PLACEMENT_3D ( 'NONE', #7114, #37998, #77012 ) ;
#65747=CARTESIAN_POINT ( 'NONE',  ( -97.59541525468981149, 48.06504152958505216, -36.50000000000000000 ) ) ;
#65752=PLANE ( 'NONE',  #70653 ) ;
#65847=LINE ( 'NONE', #12170, #79190 ) ;
#65862=DIRECTION ( 'NONE',  ( 1.000000000000000000, 0.000000000000000000, 0.000000000000000000 ) ) ;
#65879=CARTESIAN_POINT ( 'NONE',  ( -30.05470439949217365, 95.09793926796578489, 12.69393916137930667 ) ) ;
#66123=ORIENTED_EDGE ( 'NONE', *, *, #90907, .F. ) ;
#66146=AXIS2_PLACEMENT_3D ( 'NONE', #71262, #18560, #79888 ) ;
#66198=EDGE_CURVE ( 'NONE', #29349, #2126, #85983, .T. ) ;
#66210=CARTESIAN_POINT ( 'NONE',  ( -15.30390832730448913, 102.7700744756162692, 12.27820281893983356 ) ) ;
#66222=CARTESIAN_POINT ( 'NONE',  ( -31.05641173554239032, 93.49636139580346139, 11.47754913427577783 ) ) ;
#66622=FACE_OUTER_BOUND ( 'NONE', #73263, .T. ) ;
#66846=DIRECTION ( 'NONE',  ( 0.8660254037844391517, 0.4999999999999990008, 0.000000000000000000 ) ) ;
#66857=DIRECTION ( 'NONE',  ( -0.8660254037844384856, -0.5000000000000002220, 0.000000000000000000 ) ) ;
#67151=ORIENTED_EDGE ( 'NONE', *, *, #86727, .T. ) ;
#67161=EDGE_LOOP ( 'NONE', ( #1831, #59914, #99781, #36723 ) ) ;
#67162=ORIENTED_EDGE ( 'NONE', *, *, #112, .T. ) ;
#67348=CARTESIAN_POINT ( 'NONE',  ( -162.0327448629461742, 33.95614270198240803, -21.50000000000000000 ) ) ;
#67370=ORIENTED_EDGE ( 'NONE', *, *, #59302, .T. ) ;
#67375=CARTESIAN_POINT ( 'NONE',  ( -30.74362438759401428, 96.14847806106469363, 12.64899930806661033 ) ) ;
#67387=CARTESIAN_POINT ( 'NONE',  ( -107.5954152546898257, 65.38554960527383741, 36.50000000000000000 ) ) ;
#67448=CARTESIAN_POINT ( 'NONE',  ( -112.5954152546897262, 74.04580364311806306, 21.50000000000000000 ) ) ;
#67513=AXIS2_PLACEMENT_3D ( 'NONE', #89009, #74256, #59500 ) ;
#67594=CARTESIAN_POINT ( 'NONE',  ( 82.86586985908988368, 152.2544130683315871, 0.000000000000000000 ) ) ;
#67693=AXIS2_PLACEMENT_3D ( 'NONE', #32216, #85989, #86484 ) ;
#67737=VECTOR ( 'NONE', #5089, 1000.000000000000114 ) ;
#67744=VERTEX_POINT ( 'NONE', #35010 ) ;
#67809=DIRECTION ( 'NONE',  ( -7.401486830834377265E-16, 7.401486830834377265E-16, -1.000000000000000000 ) ) ;
#67832=DIRECTION ( 'NONE',  ( 0.5000000000000002220, -0.8660254037844387076, -0.000000000000000000 ) ) ;
#67897=EDGE_CURVE ( 'NONE', #86378, #94311, #72689, .T. ) ;
#67953=CARTESIAN_POINT ( 'NONE',  ( 80.86586985908986946, 155.7185146834693512, 3.300000000000006484 ) ) ;
#67975=ORIENTED_EDGE ( 'NONE', *, *, #2588, .F. ) ;
#67996=DIRECTION ( 'NONE',  ( 0.8660254037844385966, 0.4999999999999999445, 0.000000000000000000 ) ) ;
#68029=EDGE_CURVE ( 'NONE', #62277, #89481, #91870, .T. ) ;
#68037=DIRECTION ( 'NONE',  ( -0.8660254037844375974, -0.5000000000000016653, 0.000000000000000000 ) ) ;
#68155=FACE_BOUND ( 'NONE', #73599, .T. ) ;
#68159=VECTOR ( 'NONE', #38456, 1000.000000000000114 ) ;
#68265=CARTESIAN_POINT ( 'NONE',  ( -107.5954152546898257, 65.38554960527383741, 36.50000000000000000 ) ) ;
#68271=FACE_OUTER_BOUND ( 'NONE', #13483, .T. ) ;
#68328=ORIENTED_EDGE ( 'NONE', *, *, #39130, .T. ) ;
#68368=ADVANCED_FACE ( 'NONE', ( #68155, #36756, #5376 ), #5871, .T. ) ;
#68532=VERTEX_POINT ( 'NONE', #12998 ) ;
#68541=ORIENTED_EDGE ( 'NONE', *, *, #112, .F. ) ;
#68591=LINE ( 'NONE', #99514, #15879 ) ;
#68640=CIRCLE ( 'NONE', #57358, 7.273499999999997634 ) ;
#68652=DIRECTION ( 'NONE',  ( 1.000000000000000000, 0.000000000000000000, -0.000000000000000000 ) ) ;
#68784=AXIS2_PLACEMENT_3D ( 'NONE', #15354, #91924, #23457 ) ;
#68882=ADVANCED_FACE ( 'NONE', ( #45120 ), #93768, .F. ) ;
#68957=VECTOR ( 'NONE', #35251, 1000.000000000000000 ) ;
#69373=CARTESIAN_POINT ( 'NONE',  ( -32.94356256989597398, 95.08348788047962330, 10.71240442958353256 ) ) ;
#69484=DIRECTION ( 'NONE',  ( 1.000000000000000000, 0.000000000000000000, -0.000000000000000000 ) ) ;
#69665=CARTESIAN_POINT ( 'NONE',  ( -16.76269525828470464, 104.2312461070085021, 12.63376007436041171 ) ) ;
#69833=CARTESIAN_POINT ( 'NONE',  ( 82.86586985908988368, 152.2544130683315871, 0.000000000000000000 ) ) ;
#69859=DIRECTION ( 'NONE',  ( 0.5000000000000002220, -0.8660254037844387076, -0.000000000000000000 ) ) ;
#69900=EDGE_CURVE ( 'NONE', #86369, #23627, #78661, .T. ) ;
#69910=DIRECTION ( 'NONE',  ( 0.8660254037844385966, 0.4999999999999999445, 0.000000000000000000 ) ) ;
#70135=ORIENTED_EDGE ( 'NONE', *, *, #19596, .F. ) ;
#70221=VECTOR ( 'NONE', #11139, 1000.000000000000227 ) ;
#70298=CIRCLE ( 'NONE', #21790, 7.298499999999999766 ) ;
#70340=ADVANCED_FACE ( 'NONE', ( #86704 ), #62837, .T. ) ;
#70420=CARTESIAN_POINT ( 'NONE',  ( 82.93017357788667709, 175.3855496052738374, 36.50000000000000000 ) ) ;
#70485=CARTESIAN_POINT ( 'NONE',  ( -14.65312891409034535, 84.40478749174073414, 0.000000000000000000 ) ) ;
#70508=CARTESIAN_POINT ( 'NONE',  ( 77.93017357788674815, 184.0458036431181768, 30.52142883766498116 ) ) ;
#70653=AXIS2_PLACEMENT_3D ( 'NONE', #97203, #20179, #82004 ) ;
#70862=AXIS2_PLACEMENT_3D ( 'NONE', #56197, #3536, #64823 ) ;
#70923=VECTOR ( 'NONE', #53286, 1000.000000000000227 ) ;
#70939=VECTOR ( 'NONE', #55582, 1000.000000000000000 ) ;
#71003=VECTOR ( 'NONE', #94551, 1000.000000000000000 ) ;
#71262=CARTESIAN_POINT ( 'NONE',  ( -89.11465314115665137, 93.37593066204027537, -37.49999999999999289 ) ) ;
#71312=CARTESIAN_POINT ( 'NONE',  ( -112.5954152546897262, 74.04580364311806306, 21.50000000000000000 ) ) ;
#71400=LINE ( 'NONE', #32875, #52859 ) ;
#71752=ORIENTED_EDGE ( 'NONE', *, *, #88243, .T. ) ;
#71844=CARTESIAN_POINT ( 'NONE',  ( -32.57449995691604272, 93.91662174944717378, 10.44639423499586428 ) ) ;
#71981=DIRECTION ( 'NONE',  ( -0.5000000000000014433, 0.8660254037844378194, -0.000000000000000000 ) ) ;
#72115=CARTESIAN_POINT ( 'NONE',  ( -16.76269525828470464, 104.2312461070085021, 45.19948692389422717 ) ) ;
#72134=CARTESIAN_POINT ( 'NONE',  ( 80.86586985908986946, 155.7185146834693512, 0.000000000000000000 ) ) ;
#72474=DIRECTION ( 'NONE',  ( -0.000000000000000000, -0.000000000000000000, 1.000000000000000000 ) ) ;
#72476=VERTEX_POINT ( 'NONE', #98863 ) ;
#72552=AXIS2_PLACEMENT_3D ( 'NONE', #75718, #37193, #13422 ) ;
#72689=CIRCLE ( 'NONE', #38644, 7.273499999999997634 ) ;
#72840=CARTESIAN_POINT ( 'NONE',  ( -16.57839871714885760, 103.5154107798534113, 12.75852272963258471 ) ) ;
#73015=CARTESIAN_POINT ( 'NONE',  ( -30.13607937982481744, 95.41016082721114344, 12.74739955043256501 ) ) ;
#73193=EDGE_CURVE ( 'NONE', #52672, #86487, #87360, .T. ) ;
#73263=EDGE_LOOP ( 'NONE', ( #34339, #100282, #79484, #36656, #27607, #68328, #59926, #99496, #63968, #7015, #79254, #31062 ) ) ;
#73334=CARTESIAN_POINT ( 'NONE',  ( -31.22174636879925202, 93.45486797506030996, 11.33730873907181369 ) ) ;
#73464=DIRECTION ( 'NONE',  ( 0.8660254037844390407, 0.4999999999999993339, 0.000000000000000000 ) ) ;
#73474=ORIENTED_EDGE ( 'NONE', *, *, #45013, .F. ) ;
#73492=ORIENTED_EDGE ( 'NONE', *, *, #18517, .F. ) ;
#73526=EDGE_CURVE ( 'NONE', #94383, #94311, #77478, .T. ) ;
#73599=EDGE_LOOP ( 'NONE', ( #3870, #15668 ) ) ;
#73648=VERTEX_POINT ( 'NONE', #65747 ) ;
#73653=CARTESIAN_POINT ( 'NONE',  ( -19.65312891409032403, 93.06504152958505927, 0.000000000000000000 ) ) ;
#73807=CARTESIAN_POINT ( 'NONE',  ( -15.78145869460660045, 102.8555426466057838, 12.52892818809898934 ) ) ;
#73912=LINE ( 'NONE', #91134, #15919 ) ;
#73940=CARTESIAN_POINT ( 'NONE',  ( 82.86586985908988368, 152.2544130683315871, 0.000000000000000000 ) ) ;
#73976=FACE_OUTER_BOUND ( 'NONE', #98042, .T. ) ;
#73985=CARTESIAN_POINT ( 'NONE',  ( -167.0327448629461742, 42.61639673982678289, -30.52142883766498116 ) ) ;
#73992=CARTESIAN_POINT ( 'NONE',  ( 76.56683408466376761, 148.6176630683316091, 8.907468493598274475E-16 ) ) ;
#74073=AXIS2_PLACEMENT_3D ( 'NONE', #36777, #84911, #28683 ) ;
#74235=DIRECTION ( 'NONE',  ( 0.8660254037844373753, 0.5000000000000021094, 0.000000000000000000 ) ) ;
#74256=DIRECTION ( 'NONE',  ( -0.8660254037844383745, -0.5000000000000004441, 0.000000000000000000 ) ) ;
#74332=CARTESIAN_POINT ( 'NONE',  ( -13.86269525828472204, 104.0355397767245194, 10.71312146367169404 ) ) ;
#74741=CARTESIAN_POINT ( 'NONE',  ( -169.5327448629461742, 46.94652375874896677, -30.52142883766498116 ) ) ;
#74787=EDGE_CURVE ( 'NONE', #47085, #85740, #48534, .T. ) ;
#74842=ORIENTED_EDGE ( 'NONE', *, *, #39847, .T. ) ;
#74975=DIRECTION ( 'NONE',  ( -1.000000000000000000, 0.000000000000000000, -0.000000000000000000 ) ) ;
#75260=EDGE_LOOP ( 'NONE', ( #95507, #50465, #95331, #3092, #83013 ) ) ;
#75347=ORIENTED_EDGE ( 'NONE', *, *, #30973, .T. ) ;
#75422=VECTOR ( 'NONE', #52921, 1000.000000000000114 ) ;
#75563=FACE_BOUND ( 'NONE', #65266, .T. ) ;
#75718=CARTESIAN_POINT ( 'NONE',  ( -31.49356256989596758, 94.88921800892812541, 36.50000000000000000 ) ) ;
#75759=CARTESIAN_POINT ( 'NONE',  ( -16.71725632976956888, 104.6388057647513961, 12.47619570403008105 ) ) ;
#76308=ORIENTED_EDGE ( 'NONE', *, *, #73193, .F. ) ;
#76643=EDGE_CURVE ( 'NONE', #68532, #50939, #43288, .T. ) ;
#76719=ORIENTED_EDGE ( 'NONE', *, *, #58580, .F. ) ;
#76735=DIRECTION ( 'NONE',  ( -0.000000000000000000, -0.000000000000000000, 1.000000000000000000 ) ) ;
#76775=PLANE ( 'NONE',  #74073 ) ;
#76817=ORIENTED_EDGE ( 'NONE', *, *, #9759, .F. ) ;
#76895=EDGE_CURVE ( 'NONE', #56834, #50040, #68591, .T. ) ;
#77012=DIRECTION ( 'NONE',  ( -0.5000000000000002220, 0.8660254037844384856, 0.000000000000000000 ) ) ;
#77053=EDGE_CURVE ( 'NONE', #94311, #86378, #6124, .T. ) ;
#77086=FACE_BOUND ( 'NONE', #47440, .T. ) ;
#77146=AXIS2_PLACEMENT_3D ( 'NONE', #100078, #83403, #83909 ) ;
#77183=CARTESIAN_POINT ( 'NONE',  ( -97.59541525468981149, 48.06504152958505216, 36.50000000000000000 ) ) ;
#77192=ORIENTED_EDGE ( 'NONE', *, *, #77877, .F. ) ;
#77356=ORIENTED_EDGE ( 'NONE', *, *, #28818, .F. ) ;
#77374=MANIFOLD_SOLID_BREP ( 'Boss-Extrude13', #58778 ) ;
#77478=LINE ( 'NONE', #47552, #4830 ) ;
#77569=SHAPE_DEFINITION_REPRESENTATION ( #11989, #87244 ) ;
#77599=VECTOR ( 'NONE', #77910, 1000.000000000000000 ) ;
#77608=CARTESIAN_POINT ( 'NONE',  ( 85.72375369157853697, 153.9044130683316212, 0.000000000000000000 ) ) ;
#77669=EDGE_CURVE ( 'NONE', #29127, #82530, #8757, .T. ) ;
#77877=EDGE_CURVE ( 'NONE', #56899, #37919, #96654, .T. ) ;
#77883=VERTEX_POINT ( 'NONE', #79462 ) ;
#77910=DIRECTION ( 'NONE',  ( 1.716797197045744035E-15, -2.973579971575064630E-15, 1.000000000000000000 ) ) ;
#78145=CARTESIAN_POINT ( 'NONE',  ( -169.5327448629461742, 46.94652375874896677, -30.52142883766498116 ) ) ;
#78210=CARTESIAN_POINT ( 'NONE',  ( -26.40302582819689547, -15.24379406933011616, -3.684716733547464345E-15 ) ) ;
#78265=DIRECTION ( 'NONE',  ( -0.8660254037844387076, -0.5000000000000000000, 0.000000000000000000 ) ) ;
#78305=LINE ( 'NONE', #30697, #62977 ) ;
#78309=CARTESIAN_POINT ( 'NONE',  ( -89.11465314115665137, 93.37593066204027537, -37.49999999999999289 ) ) ;
#78374=FACE_OUTER_BOUND ( 'NONE', #22639, .T. ) ;
#78470=EDGE_LOOP ( 'NONE', ( #64070, #59763, #37340, #7439 ) ) ;
#78518=ORIENTED_EDGE ( 'NONE', *, *, #15300, .F. ) ;
#78661=LINE ( 'NONE', #62938, #28906 ) ;
#78724=ORIENTED_EDGE ( 'NONE', *, *, #86126, .T. ) ;
#78872=ADVANCED_FACE ( 'NONE', ( #37092 ), #59888, .F. ) ;
#79062=VERTEX_POINT ( 'NONE', #32986 ) ;
#79084=CARTESIAN_POINT ( 'NONE',  ( 92.93017357788669131, 158.0650415295850735, 36.50000000000000000 ) ) ;
#79135=ORIENTED_EDGE ( 'NONE', *, *, #44335, .F. ) ;
#79190=VECTOR ( 'NONE', #12682, 1000.000000000000000 ) ;
#79254=ORIENTED_EDGE ( 'NONE', *, *, #10174, .F. ) ;
#79423=ORIENTED_EDGE ( 'NONE', *, *, #77669, .T. ) ;
#79462=CARTESIAN_POINT ( 'NONE',  ( 77.93017357788673394, 184.0458036431182052, -30.52142883766498116 ) ) ;
#79484=ORIENTED_EDGE ( 'NONE', *, *, #41041, .T. ) ;
#79528=ADVANCED_FACE ( 'NONE', ( #93589, #78374 ), #24157, .T. ) ;
#79888=DIRECTION ( 'NONE',  ( 0.000000000000000000, 1.000000000000000000, 3.433861939970638790E-16 ) ) ;
#80132=ORIENTED_EDGE ( 'NONE', *, *, #21354, .T. ) ;
#80206=EDGE_CURVE ( 'NONE', #12458, #83357, #62470, .T. ) ;
#80228=ADVANCED_FACE ( 'NONE', ( #10307 ), #32598, .F. ) ;
#80318=AXIS2_PLACEMENT_3D ( 'NONE', #5738, #44225, #68037 ) ;
#80355=ORIENTED_EDGE ( 'NONE', *, *, #10198, .T. ) ;
#80450=VECTOR ( 'NONE', #59267, 1000.000000000000000 ) ;
#80457=CARTESIAN_POINT ( 'NONE',  ( -16.76269525828470464, 104.2312461070085021, 12.63376007436041171 ) ) ;
#80500=LINE ( 'NONE', #88614, #34662 ) ;
#80783=DIRECTION ( 'NONE',  ( -0.5000000000000003331, 0.8660254037844383745, 0.000000000000000000 ) ) ;
#80831=VECTOR ( 'NONE', #11419, 1000.000000000000114 ) ;
#80847=LINE ( 'NONE', #41269, #80831 ) ;
#80903=DIRECTION ( 'NONE',  ( -0.8660254037844363761, -0.5000000000000039968, 0.000000000000000000 ) ) ;
#80911=CARTESIAN_POINT ( 'NONE',  ( -14.09895056762408494, 105.0318923338749642, 10.41638685176045698 ) ) ;
#80963=LINE ( 'NONE', #11527, #31454 ) ;
#81018=VECTOR ( 'NONE', #56106, 1000.000000000000227 ) ;
#81173=CARTESIAN_POINT ( 'NONE',  ( -32.94356256989595977, 94.88921800892812541, 45.19948692389422717 ) ) ;
#81268=CARTESIAN_POINT ( 'NONE',  ( -112.5954152546897262, 74.04580364311806306, -21.50000000000000000 ) ) ;
#81312=ORIENTED_EDGE ( 'NONE', *, *, #93824, .F. ) ;
#81400=LINE ( 'NONE', #87540, #68957 ) ;
#81616=DIRECTION ( 'NONE',  ( 0.5000000000000001110, -0.8660254037844384856, -0.000000000000000000 ) ) ;
#81625=CARTESIAN_POINT ( 'NONE',  ( -30.49513100206280569, 95.94612159648924887, 12.72072555747216249 ) ) ;
#81646=DIRECTION ( 'NONE',  ( 6.938893903907209642E-16, -1.201851678989722492E-15, 1.000000000000000000 ) ) ;
#81678=EDGE_LOOP ( 'NONE', ( #57904, #76719, #67370, #93008 ) ) ;
#81896=FACE_OUTER_BOUND ( 'NONE', #8849, .T. ) ;
#81917=ADVANCED_FACE ( 'NONE', ( #63245 ), #6428, .F. ) ;
#81939=CARTESIAN_POINT ( 'NONE',  ( -14.12104474639061458, 103.3883419700267865, 11.22454184241338027 ) ) ;
#81964=ORIENTED_EDGE ( 'NONE', *, *, #44894, .F. ) ;
#82004=DIRECTION ( 'NONE',  ( 0.8660254037844378194, 0.5000000000000013323, 0.000000000000000000 ) ) ;
#82017=EDGE_LOOP ( 'NONE', ( #76817, #97919, #3932, #59241 ) ) ;
#82142=ORIENTED_EDGE ( 'NONE', *, *, #42846, .F. ) ;
#82515=ADVANCED_FACE ( 'NONE', ( #94265 ), #15713, .F. ) ;
#82530=VERTEX_POINT ( 'NONE', #54202 ) ;
#82563=DIRECTION ( 'NONE',  ( 1.000000000000000000, 0.000000000000000000, -0.000000000000000000 ) ) ;
#82644=CARTESIAN_POINT ( 'NONE',  ( -30.04356256989597540, 94.99361293546084539, 12.66716928022279909 ) ) ;
#82664=DIRECTION ( 'NONE',  ( 0.000000000000000000, 0.000000000000000000, 1.000000000000000000 ) ) ;
#82786=EDGE_CURVE ( 'NONE', #41262, #32844, #91128, .T. ) ;
#82850=DIRECTION ( 'NONE',  ( 0.5000000000000001110, -0.8660254037844384856, -0.000000000000000000 ) ) ;
#83013=ORIENTED_EDGE ( 'NONE', *, *, #99333, .F. ) ;
#83072=ORIENTED_EDGE ( 'NONE', *, *, #99333, .T. ) ;
#83177=ADVANCED_FACE ( 'NONE', ( #60048 ), #92494, .F. ) ;
#83219=ORIENTED_EDGE ( 'NONE', *, *, #10174, .T. ) ;
#83231=CARTESIAN_POINT ( 'NONE',  ( 82.93017357788667709, 175.3855496052738374, 36.50000000000000000 ) ) ;
#83276=EDGE_CURVE ( 'NONE', #77883, #26521, #7609, .T. ) ;
#83343=DIRECTION ( 'NONE',  ( 0.8660254037844382635, 0.5000000000000005551, 0.000000000000000000 ) ) ;
#83357=VERTEX_POINT ( 'NONE', #30520 ) ;
#83403=DIRECTION ( 'NONE',  ( -0.5000000000000014433, 0.8660254037844378194, -0.000000000000000000 ) ) ;
#83498=VECTOR ( 'NONE', #67809, 1000.000000000000000 ) ;
#83538=B_SPLINE_CURVE_WITH_KNOTS ( 'NONE', 3,
 ( #96659, #27229, #97160, #49029, #3921, #25739, #34320, #71844, #65218, #20129, #56618, #50504, #2442, #73334, #66222, #11540, #19643, #64732, #19147, #50021, #88087, #34803, #58594, #18128 ),
 .UNSPECIFIED., .F., .F.,
 ( 4, 2, 2, 2, 2, 2, 2, 2, 2, 2, 2, 4 ),
 ( 0.005192606658219600137, 0.005519221611633958260, 0.005845836565048317252, 0.006172451518462674508, 0.006499066471877033499, 0.007152296378705787910, 0.007805526285534543189, 0.008458756192363282855, 0.009111986099192019919, 0.009765216006020758718, 0.01009183095943514720, 0.01041844591284953395 ),
 .UNSPECIFIED. ) ;
#83909=DIRECTION ( 'NONE',  ( -0.8660254037844375974, -0.5000000000000016653, 0.000000000000000000 ) ) ;
#83988=CARTESIAN_POINT ( 'NONE',  ( -97.59541525468981149, 48.06504152958505216, 36.50000000000000000 ) ) ;
#84176=ORIENTED_EDGE ( 'NONE', *, *, #32666, .T. ) ;
#84328=ORIENTED_EDGE ( 'NONE', *, *, #85239, .F. ) ;
#84449=VERTEX_POINT ( 'NONE', #94604 ) ;
#84541=CARTESIAN_POINT ( 'NONE',  ( -162.0327448629461742, 33.95614270198240803, 21.50000000000000000 ) ) ;
#84745=LINE ( 'NONE', #23390, #88350 ) ;
#84872=ADVANCED_FACE ( 'NONE', ( #5800 ), #36188, .F. ) ;
#84911=DIRECTION ( 'NONE',  ( 0.5000000000000003331, -0.8660254037844385966, 8.877441173312408730E-15 ) ) ;
#85079=AXIS2_PLACEMENT_3D ( 'NONE', #96805, #65356, #66846 ) ;
#85188=DIRECTION ( 'NONE',  ( -0.8660254037844384856, -0.5000000000000002220, 0.000000000000000000 ) ) ;
#85196=VECTOR ( 'NONE', #81616, 1000.000000000000227 ) ;
#85239=EDGE_CURVE ( 'NONE', #2126, #19964, #65001, .T. ) ;
#85273=CARTESIAN_POINT ( 'NONE',  ( -112.5954152546897120, 74.04580364311804885, 30.52142883766498116 ) ) ;
#85367=CARTESIAN_POINT ( 'NONE',  ( 92.93017357788669131, 158.0650415295850735, 36.50000000000000000 ) ) ;
#85513=STYLED_ITEM('',(#100310),#77374);
#85740=VERTEX_POINT ( 'NONE', #83988 ) ;
#85835=DIRECTION ( 'NONE',  ( 0.000000000000000000, 0.000000000000000000, 1.000000000000000000 ) ) ;
#85983=LINE ( 'NONE', #8417, #71003 ) ;
#85989=DIRECTION ( 'NONE',  ( 0.000000000000000000, 0.000000000000000000, -1.000000000000000000 ) ) ;
#86126=EDGE_CURVE ( 'NONE', #52672, #10803, #30375, .T. ) ;
#86138=DIRECTION ( 'NONE',  ( 0.5000000000000003331, -0.8660254037844385966, 8.877441173312408730E-15 ) ) ;
#86164=EDGE_LOOP ( 'NONE', ( #65036, #99150, #67162, #2371 ) ) ;
#86231=ORIENTED_EDGE ( 'NONE', *, *, #77053, .F. ) ;
#86286=EDGE_CURVE ( 'NONE', #44968, #43056, #89281, .T. ) ;
#86369=VERTEX_POINT ( 'NONE', #78309 ) ;
#86378=VERTEX_POINT ( 'NONE', #11912 ) ;
#86395=B_SPLINE_CURVE_WITH_KNOTS ( 'NONE', 3,
 ( #80457, #41901, #11529, #50008, #58101, #72840, #12018, #89083, #19632, #65207, #96148, #50492, #73807, #35298, #66210, #20118, #50989, #81939, #12517, #43389, #74332, #4920 ),
 .UNSPECIFIED., .F., .F.,
 ( 4, 2, 2, 2, 2, 2, 2, 2, 2, 2, 4 ),
 ( 0.005247342714528634502, 0.005571968392429927155, 0.005896594070331220676, 0.006221219748232513329, 0.006545845426133806849, 0.006870471104035099502, 0.007195096781936393023, 0.007844348137738960114, 0.009142850849344096031, 0.009792102205146660521, 0.01044135356094922501 ),
 .UNSPECIFIED. ) ;
#86475=ORIENTED_EDGE ( 'NONE', *, *, #97239, .T. ) ;
#86484=DIRECTION ( 'NONE',  ( -1.000000000000000000, 0.000000000000000000, -0.000000000000000000 ) ) ;
#86487=VERTEX_POINT ( 'NONE', #29099 ) ;
#86517=CARTESIAN_POINT ( 'NONE',  ( 77.93017357788673394, 184.0458036431182052, -21.50000000000000000 ) ) ;
#86650=ORIENTED_EDGE ( 'NONE', *, *, #50936, .T. ) ;
#86704=FACE_OUTER_BOUND ( 'NONE', #36854, .T. ) ;
#86714=ORIENTED_EDGE ( 'NONE', *, *, #74787, .F. ) ;
#86727=EDGE_CURVE ( 'NONE', #57005, #29127, #16871, .T. ) ;
#86752=DIRECTION ( 'NONE',  ( -0.8660254037844385966, -0.5000000000000001110, 0.000000000000000000 ) ) ;
#86791=DIRECTION ( 'NONE',  ( 0.8660254037844382635, 0.5000000000000005551, 0.000000000000000000 ) ) ;
#86823=ORIENTED_EDGE ( 'NONE', *, *, #18517, .T. ) ;
#86850=VECTOR ( 'NONE', #60756, 1000.000000000000000 ) ;
#86890=CIRCLE ( 'NONE', #5975, 3.300000000000010925 ) ;
#87068=( NAMED_UNIT ( * ) SI_UNIT ( $, .STERADIAN. ) SOLID_ANGLE_UNIT ( ) );
#87145=ORIENTED_EDGE ( 'NONE', *, *, #60007, .F. ) ;
#87244=SHAPE_REPRESENTATION ( 'Upper Movable Jaw Swivel Body', ( #68784 ), #36458 ) ;
#87303=ORIENTED_EDGE ( 'NONE', *, *, #22835, .T. ) ;
#87360=LINE ( 'NONE', #56858, #22526 ) ;
#87540=CARTESIAN_POINT ( 'NONE',  ( -112.5954152546897262, 74.04580364311806306, -21.50000000000000000 ) ) ;
#87689=ADVANCED_FACE ( 'NONE', ( #2563 ), #57229, .F. ) ;
#87741=CARTESIAN_POINT ( 'NONE',  ( 77.93017357788673394, 184.0458036431182052, -21.50000000000000000 ) ) ;
#87868=DIRECTION ( 'NONE',  ( -0.000000000000000000, -0.000000000000000000, 1.000000000000000000 ) ) ;
#88019=CARTESIAN_POINT ( 'NONE',  ( -16.45508872280957036, 105.1413016814280894, 12.14368461262158583 ) ) ;
#88064=( NAMED_UNIT ( * ) PLANE_ANGLE_UNIT ( ) SI_UNIT ( $, .RADIAN. ) );
#88087=CARTESIAN_POINT ( 'NONE',  ( -30.09721120228516966, 94.48592239574253426, 12.47173656650774731 ) ) ;
#88243=EDGE_CURVE ( 'NONE', #91866, #91566, #39157, .T. ) ;
#88245=EDGE_CURVE ( 'NONE', #85740, #73648, #30592, .T. ) ;
#88350=VECTOR ( 'NONE', #23896, 1000.000000000000114 ) ;
#88356=CARTESIAN_POINT ( 'NONE',  ( -89.11465314115667979, 93.37593066204033221, -30.52142883766496695 ) ) ;
#88382=ORIENTED_EDGE ( 'NONE', *, *, #54455, .T. ) ;
#88614=CARTESIAN_POINT ( 'NONE',  ( -115.0954152546898257, 78.37593066204033221, -30.52142883766496695 ) ) ;
#88629=ADVANCED_FACE ( 'NONE', ( #5067 ), #34948, .T. ) ;
#88632=ORIENTED_EDGE ( 'NONE', *, *, #63428, .T. ) ;
#88768=VECTOR ( 'NONE', #86791, 1000.000000000000114 ) ;
#88861=VERTEX_POINT ( 'NONE', #8555 ) ;
#88878=CARTESIAN_POINT ( 'NONE',  ( 82.93017357788673394, 175.3855496052738374, -21.50000000000000000 ) ) ;
#89009=CARTESIAN_POINT ( 'NONE',  ( 92.93017357788669131, 158.0650415295850735, 36.50000000000000000 ) ) ;
#89032=CARTESIAN_POINT ( 'NONE',  ( -14.04074883167679566, 104.9358293318823456, 10.41391694355407083 ) ) ;
#89083=CARTESIAN_POINT ( 'NONE',  ( -16.38799186764660831, 103.2525231626253657, 12.73778727189863780 ) ) ;
#89237=CARTESIAN_POINT ( 'NONE',  ( -106.6146531411566798, 123.6868197944956620, 37.50000000000002132 ) ) ;
#89277=CARTESIAN_POINT ( 'NONE',  ( -115.0954152546897973, 78.37593066204027537, 37.50000000000002132 ) ) ;
#89281=CIRCLE ( 'NONE', #24486, 7.298499999999999766 ) ;
#89400=DIRECTION ( 'NONE',  ( 0.5000000000000002220, -0.8660254037844387076, -0.000000000000000000 ) ) ;
#89401=CARTESIAN_POINT ( 'NONE',  ( -106.6146531411567224, 123.6868197944957188, -37.49999999999997868 ) ) ;
#89402=DIRECTION ( 'NONE',  ( -0.8660254037844387076, -0.5000000000000000000, 0.000000000000000000 ) ) ;
#89481=VERTEX_POINT ( 'NONE', #88878 ) ;
#89514=CARTESIAN_POINT ( 'NONE',  ( -115.0954152546897973, 78.37593066204027537, -37.49999999999999289 ) ) ;
#89533=AXIS2_PLACEMENT_3D ( 'NONE', #56851, #85835, #2180 ) ;
#89665=AXIS2_PLACEMENT_3D ( 'NONE', #84541, #15085, #82563 ) ;
#89683=PRODUCT ( 'Upper Movable Jaw Swivel Body', 'Upper Movable Jaw Swivel Body', '', ( #60829 ) ) ;
#89878=EDGE_CURVE ( 'NONE', #19964, #91708, #56083, .T. ) ;
#89985=CARTESIAN_POINT ( 'NONE',  ( -13.86269525828471849, 104.3301040240179418, 10.56608444709879713 ) ) ;
#90102=ORIENTED_EDGE ( 'NONE', *, *, #86126, .F. ) ;
#90141=AXIS2_PLACEMENT_3D ( 'NONE', #54310, #61918, #93372 ) ;
#90293=AXIS2_PLACEMENT_3D ( 'NONE', #70485, #96328, #35482 ) ;
#90411=AXIS2_PLACEMENT_3D ( 'NONE', #64347, #95311, #85188 ) ;
#90481=ORIENTED_EDGE ( 'NONE', *, *, #80206, .F. ) ;
#90748=LINE ( 'NONE', #67387, #80450 ) ;
#90768=CARTESIAN_POINT ( 'NONE',  ( 77.93017357788674815, 184.0458036431181768, 30.52142883766498116 ) ) ;
#90907=EDGE_CURVE ( 'NONE', #47085, #52672, #90748, .T. ) ;
#91128=LINE ( 'NONE', #30790, #16182 ) ;
#91134=CARTESIAN_POINT ( 'NONE',  ( -115.0954152546898257, 78.37593066204033221, -30.52142883766496695 ) ) ;
#91252=EDGE_CURVE ( 'NONE', #50939, #68532, #64282, .T. ) ;
#91475=CARTESIAN_POINT ( 'NONE',  ( -15.31269525828471068, 104.2312461070085021, 45.19948692389422717 ) ) ;
#91491=AXIS2_PLACEMENT_3D ( 'NONE', #95993, #42226, #58423 ) ;
#91499=DIRECTION ( 'NONE',  ( 1.000000000000000000, 0.000000000000000000, 0.000000000000000000 ) ) ;
#91566=VERTEX_POINT ( 'NONE', #63175 ) ;
#91600=DIRECTION ( 'NONE',  ( -0.5000000000000005551, 0.8660254037844384856, 0.000000000000000000 ) ) ;
#91708=VERTEX_POINT ( 'NONE', #8976 ) ;
#91746=EDGE_LOOP ( 'NONE', ( #24373, #87145 ) ) ;
#91836=VERTEX_POINT ( 'NONE', #86517 ) ;
#91848=VECTOR ( 'NONE', #43082, 1000.000000000000000 ) ;
#91866=VERTEX_POINT ( 'NONE', #31732 ) ;
#91870=LINE ( 'NONE', #53316, #35474 ) ;
#91924=DIRECTION ( 'NONE',  ( 0.000000000000000000, 0.000000000000000000, 1.000000000000000000 ) ) ;
#92068=ORIENTED_EDGE ( 'NONE', *, *, #61063, .T. ) ;
#92228=CARTESIAN_POINT ( 'NONE',  ( -107.5954152546897262, 65.38554960527366688, 21.50000000000000000 ) ) ;
#92494=CYLINDRICAL_SURFACE ( 'NONE', #11374, 1.449999999999993072 ) ;
#92678=ORIENTED_EDGE ( 'NONE', *, *, #97239, .F. ) ;
#92716=ORIENTED_EDGE ( 'NONE', *, *, #42846, .T. ) ;
#92812=VECTOR ( 'NONE', #34802, 1000.000000000000227 ) ;
#93008=ORIENTED_EDGE ( 'NONE', *, *, #76643, .T. ) ;
#93009=LINE ( 'NONE', #30691, #14147 ) ;
#93056=ORIENTED_EDGE ( 'NONE', *, *, #45138, .T. ) ;
#93323=EDGE_CURVE ( 'NONE', #99384, #29626, #83538, .T. ) ;
#93372=DIRECTION ( 'NONE',  ( 1.000000000000000000, 0.000000000000000000, -0.000000000000000000 ) ) ;
#93589=FACE_BOUND ( 'NONE', #33448, .T. ) ;
#93768=PLANE ( 'NONE',  #97068 ) ;
#93824=EDGE_CURVE ( 'NONE', #24620, #91836, #56238, .T. ) ;
#93846=CARTESIAN_POINT ( 'NONE',  ( -30.04356256989558815, 94.88921800892795488, 12.63376007436073323 ) ) ;
#93996=UNCERTAINTY_MEASURE_WITH_UNIT (LENGTH_MEASURE( 1.000000000000000082E-05 ), #678, 'distance_accuracy_value', 'NONE');
#94186=CARTESIAN_POINT ( 'NONE',  ( 82.86586985908988368, 152.2544130683315871, 0.000000000000000000 ) ) ;
#94265=FACE_OUTER_BOUND ( 'NONE', #82017, .T. ) ;
#94311=VERTEX_POINT ( 'NONE', #12050 ) ;
#94383=VERTEX_POINT ( 'NONE', #13058 ) ;
#94551=DIRECTION ( 'NONE',  ( 4.546899780356472071E-16, -9.093799560712944142E-16, 1.000000000000000000 ) ) ;
#94584=EDGE_LOOP ( 'NONE', ( #59366, #99036, #59999, #25232 ) ) ;
#94596=EDGE_CURVE ( 'NONE', #46799, #29349, #52400, .T. ) ;
#94604=CARTESIAN_POINT ( 'NONE',  ( 82.93017357788667709, 175.3855496052738374, 36.50000000000000000 ) ) ;
#94636=( LENGTH_UNIT ( ) NAMED_UNIT ( * ) SI_UNIT ( .MILLI., .METRE. ) );
#94639=CIRCLE ( 'NONE', #47651, 14.99999999999968381 ) ;
#94779=CARTESIAN_POINT ( 'NONE',  ( -31.49356256989596758, 94.88921800892812541, 45.19948692389422717 ) ) ;
#94941=ORIENTED_EDGE ( 'NONE', *, *, #76895, .T. ) ;
#95140=CARTESIAN_POINT ( 'NONE',  ( -89.11465314115665137, 93.37593066204027537, 30.52142883766497405 ) ) ;
#95193=AXIS2_PLACEMENT_3D ( 'NONE', #62882, #32500, #86752 ) ;
#95215=EDGE_CURVE ( 'NONE', #20667, #83357, #40998, .T. ) ;
#95266=AXIS2_PLACEMENT_3D ( 'NONE', #3372, #34734, #80903 ) ;
#95311=DIRECTION ( 'NONE',  ( -0.5000000000000003331, 0.8660254037844385966, 1.011061903669573814E-15 ) ) ;
#95331=ORIENTED_EDGE ( 'NONE', *, *, #16721, .F. ) ;
#95507=ORIENTED_EDGE ( 'NONE', *, *, #10198, .F. ) ;
#95609=CARTESIAN_POINT ( 'NONE',  ( -14.65312891409034535, 84.40478749174073414, 0.000000000000000000 ) ) ;
#95993=CARTESIAN_POINT ( 'NONE',  ( -14.65312891409034535, 84.40478749174073414, 0.000000000000000000 ) ) ;
#96148=CARTESIAN_POINT ( 'NONE',  ( -16.05822657194880421, 102.9833706691409105, 12.64279042072237580 ) ) ;
#96193=ORIENTED_EDGE ( 'NONE', *, *, #19596, .T. ) ;
#96223=LINE ( 'NONE', #68265, #62369 ) ;
#96254=CARTESIAN_POINT ( 'NONE',  ( 80.00798602660123038, 150.6044130683315814, 4.041334437186263538E-16 ) ) ;
#96317=VECTOR ( 'NONE', #37051, 1000.000000000000000 ) ;
#96328=DIRECTION ( 'NONE',  ( 0.5000000000000014433, -0.8660254037844379305, 0.000000000000000000 ) ) ;
#96600=CARTESIAN_POINT ( 'NONE',  ( -13.86269525828469895, 104.2312461070084879, 10.61543114587583148 ) ) ;
#96654=LINE ( 'NONE', #10026, #98496 ) ;
#96659=CARTESIAN_POINT ( 'NONE',  ( -32.94356256989595977, 94.88921800892812541, 10.61543114587583503 ) ) ;
#96769=AXIS2_PLACEMENT_3D ( 'NONE', #100191, #14075, #99187 ) ;
#96784=( GEOMETRIC_REPRESENTATION_CONTEXT ( 3 ) GLOBAL_UNCERTAINTY_ASSIGNED_CONTEXT ( ( #2784 ) ) GLOBAL_UNIT_ASSIGNED_CONTEXT ( ( #94636, #88064, #87068 ) ) REPRESENTATION_CONTEXT ( 'NONE', 'WORKASPACE' ) );
#96805=CARTESIAN_POINT ( 'NONE',  ( 82.86586985908988368, 152.2544130683315871, 0.000000000000000000 ) ) ;
#97068=AXIS2_PLACEMENT_3D ( 'NONE', #70420, #24326, #69910 ) ;
#97160=CARTESIAN_POINT ( 'NONE',  ( -32.93344297370182971, 94.68900127417109047, 10.52354740462235760 ) ) ;
#97203=CARTESIAN_POINT ( 'NONE',  ( -14.65312891409034535, 84.40478749174073414, 0.000000000000000000 ) ) ;
#97239=EDGE_CURVE ( 'NONE', #79062, #57005, #80500, .T. ) ;
#97288=FACE_OUTER_BOUND ( 'NONE', #29833, .T. ) ;
#97706=ORIENTED_EDGE ( 'NONE', *, *, #95215, .F. ) ;
#97854=EDGE_CURVE ( 'NONE', #88861, #94383, #68640, .T. ) ;
#97899=DIRECTION ( 'NONE',  ( 4.546899780356472071E-16, -9.093799560712944142E-16, 1.000000000000000000 ) ) ;
#97919=ORIENTED_EDGE ( 'NONE', *, *, #80206, .T. ) ;
#98042=EDGE_LOOP ( 'NONE', ( #44647, #18579 ) ) ;
#98061=CARTESIAN_POINT ( 'NONE',  ( -16.06007122719572777, 105.4852662834641990, 11.75378467557247397 ) ) ;
#98301=CARTESIAN_POINT ( 'NONE',  ( -30.93189967759662196, 96.24030206069060966, 12.57434963852382559 ) ) ;
#98306=EDGE_CURVE ( 'NONE', #43056, #44968, #70298, .T. ) ;
#98400=ORIENTED_EDGE ( 'NONE', *, *, #54455, .F. ) ;
#98453=DIRECTION ( 'NONE',  ( 0.8660254037844390407, 0.4999999999999993339, 0.000000000000000000 ) ) ;
#98496=VECTOR ( 'NONE', #41910, 1000.000000000000000 ) ;
#98527=ORIENTED_EDGE ( 'NONE', *, *, #61063, .F. ) ;
#98595=CARTESIAN_POINT ( 'NONE',  ( 0.000000000000000000, 0.000000000000000000, 36.50000000000000000 ) ) ;
#98697=EDGE_LOOP ( 'NONE', ( #14906, #76308, #66123, #44314 ) ) ;
#98723=DIRECTION ( 'NONE',  ( -3.977257660627182967E-15, 7.954515321254365934E-15, 1.000000000000000000 ) ) ;
#98811=EDGE_CURVE ( 'NONE', #37839, #67744, #99372, .T. ) ;
#98863=CARTESIAN_POINT ( 'NONE',  ( 78.00798602660121617, 154.0685146834693171, 4.041334437186263538E-16 ) ) ;
#98918=CARTESIAN_POINT ( 'NONE',  ( 76.54518344956915143, 148.6051630683315921, 8.938084663576957867E-16 ) ) ;
#98986=VERTEX_POINT ( 'NONE', #34937 ) ;
#99036=ORIENTED_EDGE ( 'NONE', *, *, #18282, .T. ) ;
#99041=ADVANCED_FACE ( 'NONE', ( #57238 ), #65349, .F. ) ;
#99085=DIRECTION ( 'NONE',  ( -0.000000000000000000, -0.000000000000000000, 1.000000000000000000 ) ) ;
#99117=CARTESIAN_POINT ( 'NONE',  ( 82.86586985908988368, 152.2544130683315871, 0.000000000000000000 ) ) ;
#99150=ORIENTED_EDGE ( 'NONE', *, *, #17424, .F. ) ;
#99187=DIRECTION ( 'NONE',  ( 0.8660254037844382635, 0.5000000000000005551, 0.000000000000000000 ) ) ;
#99194=DIRECTION ( 'NONE',  ( 0.5000000000000006661, -0.8660254037844383745, 0.000000000000000000 ) ) ;
#99200=DIRECTION ( 'NONE',  ( -0.8660254037844385966, -0.4999999999999999445, 0.000000000000000000 ) ) ;
#99216=EDGE_CURVE ( 'NONE', #37919, #86487, #50308, .T. ) ;
#99333=EDGE_CURVE ( 'NONE', #79062, #2126, #54787, .T. ) ;
#99372=LINE ( 'NONE', #28970, #96317 ) ;
#99384=VERTEX_POINT ( 'NONE', #107 ) ;
#99432=ORIENTED_EDGE ( 'NONE', *, *, #89878, .T. ) ;
#99496=ORIENTED_EDGE ( 'NONE', *, *, #77877, .T. ) ;
#99514=CARTESIAN_POINT ( 'NONE',  ( -1.662747857324054612, 91.90478749174060624, 1.836970198720990540E-15 ) ) ;
#99710=VECTOR ( 'NONE', #76735, 1000.000000000000000 ) ;
#99781=ORIENTED_EDGE ( 'NONE', *, *, #62129, .F. ) ;
#99812=CONICAL_SURFACE ( 'NONE', #85079, 7.298499999999999766, 0.7853981633976494514 ) ;
#99843=CARTESIAN_POINT ( 'NONE',  ( -15.31269525828471068, 104.2312461070085021, 45.19948692389422717 ) ) ;
#99859=DIRECTION ( 'NONE',  ( -0.5000000000000002220, 0.8660254037844385966, 0.000000000000000000 ) ) ;
#99966=DIRECTION ( 'NONE',  ( -0.8660254037844384856, -0.5000000000000002220, 0.000000000000000000 ) ) ;
#100007=DIRECTION ( 'NONE',  ( -0.5000000000000014433, 0.8660254037844379305, -0.000000000000000000 ) ) ;
#100051=ORIENTED_EDGE ( 'NONE', *, *, #98306, .T. ) ;
#100078=CARTESIAN_POINT ( 'NONE',  ( -14.65312891409034535, 84.40478749174073414, 0.000000000000000000 ) ) ;
#100191=CARTESIAN_POINT ( 'NONE',  ( -167.0327448629461742, 42.61639673982678289, 21.50000000000000000 ) ) ;
#100261=DIRECTION ( 'NONE',  ( 0.5000000000000001110, -0.8660254037844384856, -0.000000000000000000 ) ) ;
#100282=ORIENTED_EDGE ( 'NONE', *, *, #31149, .F. ) ;
#100304=COLOUR_RGB('Dark Blue',0.08,0.2,0.34);
#100305=FILL_AREA_STYLE_COLOUR('',#100304);
#100306=FILL_AREA_STYLE('',(#100305));
#100307=SURFACE_STYLE_FILL_AREA(#100306);
#100308=SURFACE_SIDE_STYLE('',(#100307));
#100309=SURFACE_STYLE_USAGE(.BOTH.,#100308);
#100310=PRESENTATION_STYLE_ASSIGNMENT((#100309));
ENDSEC;
END-ISO-10303-21;
